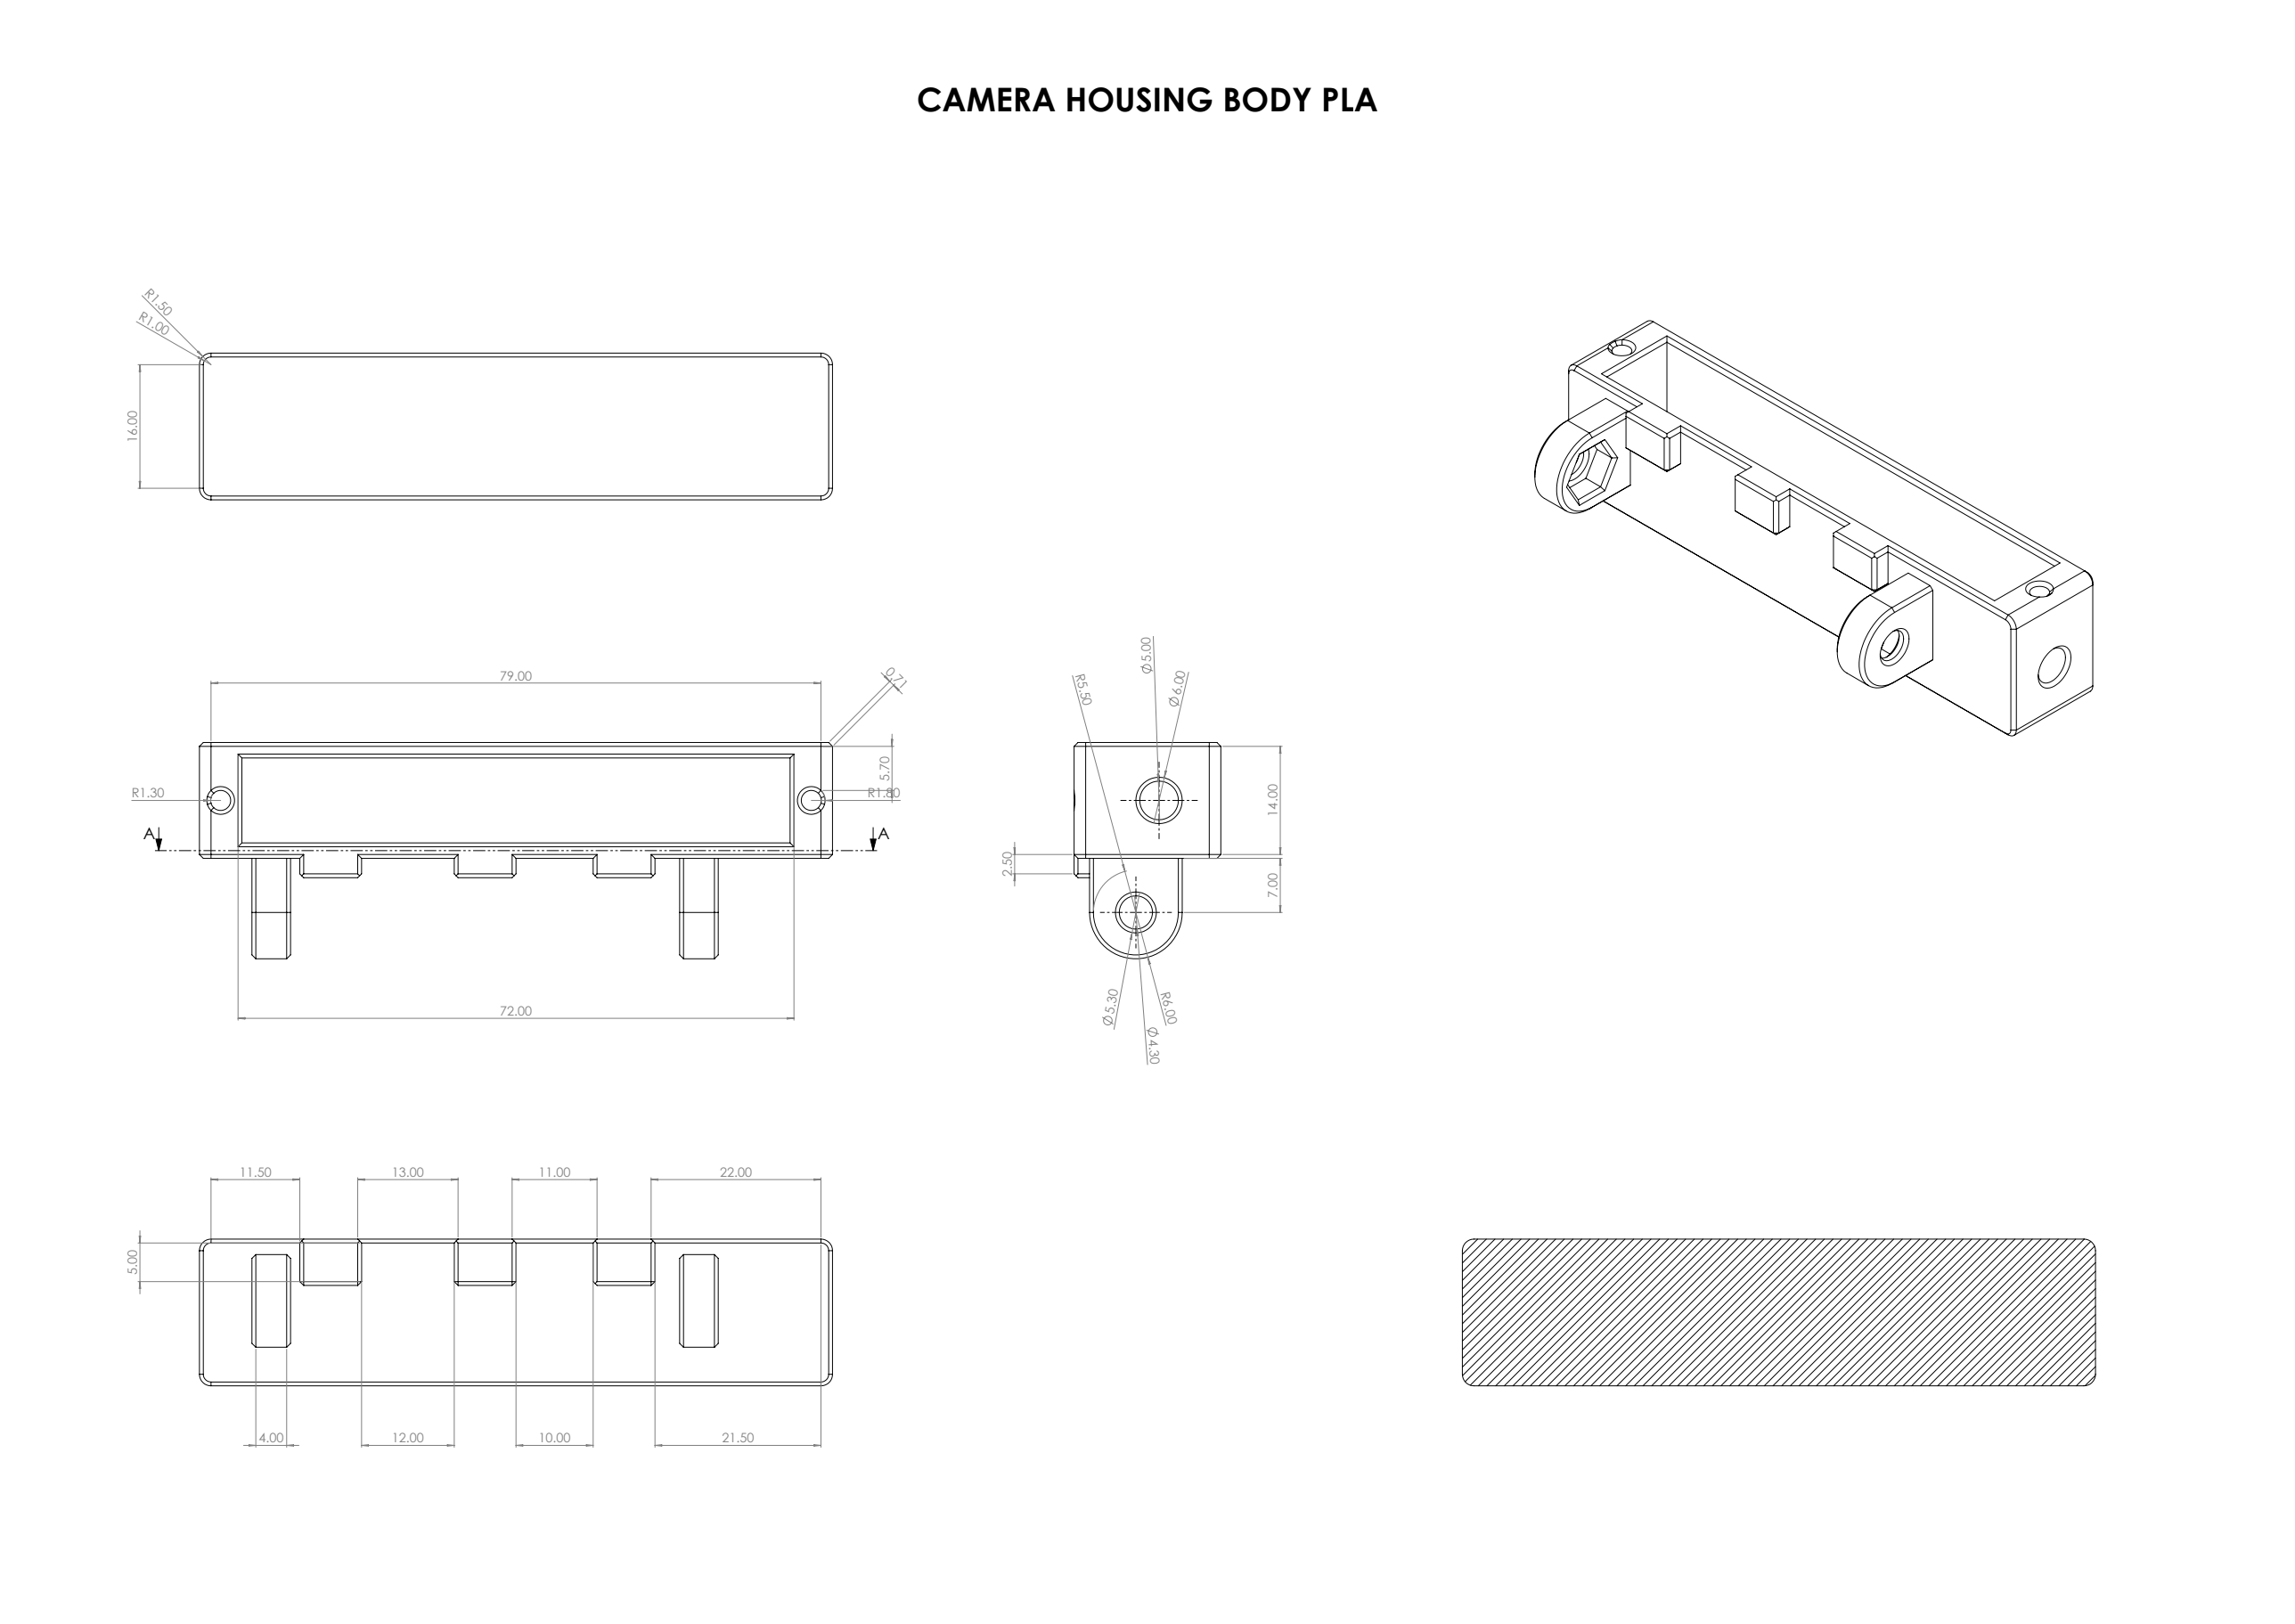
ISO-10303-21;
HEADER;
/* Generated by software containing ST-Developer
 * from STEP Tools, Inc. (www.steptools.com) 
 */

FILE_DESCRIPTION(
/* description */ (''),
/* implementation_level */ '2;1');

FILE_NAME(
/* name */ '03_Camera_Housing_Body_PLA.step',
/* time_stamp */ '2026-10-21T02:01:14-07:00',
/* author */ (''),
/* organization */ (''),
/* preprocessor_version */ 'ST-DEVELOPER v20.2',
/* originating_system */ 'Autodesk Translation Framework v15.15.0.0',
/* authorisation */ '');

FILE_SCHEMA (('AUTOMOTIVE_DESIGN { 1 0 10303 214 3 1 1 }'));
ENDSEC;

DATA;
#10=MECHANICAL_DESIGN_GEOMETRIC_PRESENTATION_REPRESENTATION('',(#616),#37181);
#105=B_SPLINE_SURFACE_WITH_KNOTS('',3,3,((#21181,#21182,#21183,#21184,#21185,
#21186),(#21187,#21188,#21189,#21190,#21191,#21192),(#21193,#21194,#21195,
#21196,#21197,#21198),(#21199,#21200,#21201,#21202,#21203,#21204)),
 .UNSPECIFIED.,.F.,.F.,.F.,(4,4),(4,2,4),(0.,1.),(0.268796457448958,0.30404357328347,
0.339290689117984),.UNSPECIFIED.);
#106=B_SPLINE_SURFACE_WITH_KNOTS('',3,3,((#21223,#21224,#21225,#21226),
(#21227,#21228,#21229,#21230),(#21231,#21232,#21233,#21234),(#21235,#21236,
#21237,#21238)),.UNSPECIFIED.,.F.,.F.,.F.,(4,4),(4,4),(0.,1.),(0.278246822734795,
0.803148805386868),.UNSPECIFIED.);
#107=B_SPLINE_SURFACE_WITH_KNOTS('',3,3,((#21243,#21244,#21245,#21246),
(#21247,#21248,#21249,#21250),(#21251,#21252,#21253,#21254),(#21255,#21256,
#21257,#21258)),.UNSPECIFIED.,.F.,.F.,.F.,(4,4),(4,4),(0.,1.),(-0.803148805386867,
-0.278246822734795),.UNSPECIFIED.);
#108=B_SPLINE_SURFACE_WITH_KNOTS('',3,3,((#21267,#21268,#21269,#21270,#21271,
#21272),(#21273,#21274,#21275,#21276,#21277,#21278),(#21279,#21280,#21281,
#21282,#21283,#21284),(#21285,#21286,#21287,#21288,#21289,#21290)),
 .UNSPECIFIED.,.F.,.F.,.F.,(4,4),(4,2,4),(0.,1.),(0.268796457448958,0.304043573283469,
0.33929068911798),.UNSPECIFIED.);
#109=B_SPLINE_SURFACE_WITH_KNOTS('',3,3,((#21310,#21311,#21312,#21313),
(#21314,#21315,#21316,#21317),(#21318,#21319,#21320,#21321),(#21322,#21323,
#21324,#21325)),.UNSPECIFIED.,.F.,.F.,.F.,(4,4),(4,4),(0.,1.),(-2.86334583085503,
-2.33844384820293),.UNSPECIFIED.);
#110=B_SPLINE_SURFACE_WITH_KNOTS('',3,3,((#21330,#21331,#21332,#21333),
(#21334,#21335,#21336,#21337),(#21338,#21339,#21340,#21341),(#21342,#21343,
#21344,#21345)),.UNSPECIFIED.,.F.,.F.,.F.,(4,4),(4,4),(0.,1.),(-3.94474145897665,
-3.41983947632457),.UNSPECIFIED.);
#128=B_SPLINE_CURVE_WITH_KNOTS('',3,(#21070,#21071,#21072,#21073),
 .UNSPECIFIED.,.F.,.F.,(4,4),(0.278246822734795,0.803148805386867),
 .UNSPECIFIED.);
#129=B_SPLINE_CURVE_WITH_KNOTS('',3,(#21075,#21076,#21077,#21078,#21079,
#21080),.UNSPECIFIED.,.F.,.F.,(4,2,4),(-0.339290689117984,-0.30404357328347,
-0.268796457448958),.UNSPECIFIED.);
#130=B_SPLINE_CURVE_WITH_KNOTS('',3,(#21081,#21082,#21083,#21084),
 .UNSPECIFIED.,.F.,.F.,(4,4),(-0.803148805386868,-0.278246822734795),
 .UNSPECIFIED.);
#131=B_SPLINE_CURVE_WITH_KNOTS('',3,(#21159,#21160,#21161,#21162),
 .UNSPECIFIED.,.F.,.F.,(4,4),(3.41983947632457,3.94474145897665),
 .UNSPECIFIED.);
#132=B_SPLINE_CURVE_WITH_KNOTS('',3,(#21164,#21165,#21166,#21167,#21168,
#21169),.UNSPECIFIED.,.F.,.F.,(4,2,4),(-0.33929068911798,-0.304043573283469,
-0.268796457448958),.UNSPECIFIED.);
#133=B_SPLINE_CURVE_WITH_KNOTS('',3,(#21170,#21171,#21172,#21173),
 .UNSPECIFIED.,.F.,.F.,(4,4),(2.33844384820293,2.86334583085503),
 .UNSPECIFIED.);
#134=B_SPLINE_CURVE_WITH_KNOTS('',3,(#21209,#21210,#21211,#21212,#21213,
#21214),.UNSPECIFIED.,.F.,.F.,(4,2,4),(0.268796457448958,0.30404357328347,
0.339290689117984),.UNSPECIFIED.);
#135=B_SPLINE_CURVE_WITH_KNOTS('',3,(#21239,#21240,#21241,#21242),
 .UNSPECIFIED.,.F.,.F.,(4,4),(0.278246822734795,0.803148805386868),
 .UNSPECIFIED.);
#136=B_SPLINE_CURVE_WITH_KNOTS('',3,(#21259,#21260,#21261,#21262),
 .UNSPECIFIED.,.F.,.F.,(4,4),(-0.803148805386867,-0.278246822734795),
 .UNSPECIFIED.);
#137=B_SPLINE_CURVE_WITH_KNOTS('',3,(#21296,#21297,#21298,#21299),
 .UNSPECIFIED.,.F.,.F.,(4,4),(0.268796457448958,0.304043573283469),
 .UNSPECIFIED.);
#138=B_SPLINE_CURVE_WITH_KNOTS('',3,(#21300,#21301,#21302,#21303),
 .UNSPECIFIED.,.F.,.F.,(4,4),(0.304043573283469,0.33929068911798),
 .UNSPECIFIED.);
#139=B_SPLINE_CURVE_WITH_KNOTS('',3,(#21326,#21327,#21328,#21329),
 .UNSPECIFIED.,.F.,.F.,(4,4),(-2.86334583085503,-2.33844384820293),
 .UNSPECIFIED.);
#140=B_SPLINE_CURVE_WITH_KNOTS('',3,(#21346,#21347,#21348,#21349),
 .UNSPECIFIED.,.F.,.F.,(4,4),(-3.94474145897665,-3.41983947632457),
 .UNSPECIFIED.);
#590=SHAPE_REPRESENTATION_RELATIONSHIP('SRR','None',#37240,#603);
#603=ADVANCED_BREP_SHAPE_REPRESENTATION('',(#629),#37170);
#616=STYLED_ITEM('',(#37352),#629);
#629=MANIFOLD_SOLID_BREP('Body1',#14778);
#654=FACE_BOUND('',#2365,.T.);
#655=FACE_BOUND('',#2382,.T.);
#656=FACE_BOUND('',#2386,.T.);
#657=FACE_BOUND('',#2389,.T.);
#658=FACE_BOUND('',#2401,.T.);
#659=FACE_BOUND('',#2415,.T.);
#660=FACE_BOUND('',#2446,.T.);
#661=FACE_BOUND('',#2457,.T.);
#662=FACE_BOUND('',#2484,.T.);
#663=FACE_BOUND('',#2485,.T.);
#664=FACE_BOUND('',#2502,.T.);
#708=CYLINDRICAL_SURFACE('',#15144,6.);
#709=CYLINDRICAL_SURFACE('',#15158,6.);
#710=CYLINDRICAL_SURFACE('',#15171,2.15);
#711=CYLINDRICAL_SURFACE('',#15177,2.15);
#712=CYLINDRICAL_SURFACE('',#15257,1.5);
#713=CYLINDRICAL_SURFACE('',#15261,1.5);
#714=CYLINDRICAL_SURFACE('',#15288,1.5);
#715=CYLINDRICAL_SURFACE('',#15290,1.5);
#716=CYLINDRICAL_SURFACE('',#15299,1.3);
#717=CYLINDRICAL_SURFACE('',#15303,1.3);
#718=CYLINDRICAL_SURFACE('',#15307,2.5);
#1019=CIRCLE('',#15140,5.5);
#1020=CIRCLE('',#15141,6.);
#1021=CIRCLE('',#15145,6.);
#1022=CIRCLE('',#15149,5.5);
#1023=CIRCLE('',#15154,5.5);
#1024=CIRCLE('',#15155,6.);
#1025=CIRCLE('',#15159,6.);
#1026=CIRCLE('',#15169,2.65);
#1027=CIRCLE('',#15170,2.15);
#1028=CIRCLE('',#15172,2.15);
#1029=CIRCLE('',#15175,2.65);
#1030=CIRCLE('',#15176,2.15);
#1031=CIRCLE('',#15178,2.15);
#1032=CIRCLE('',#15181,2.65);
#1033=CIRCLE('',#15193,2.65);
#1034=CIRCLE('',#15197,5.5);
#1035=CIRCLE('',#15239,1.8);
#1036=CIRCLE('',#15240,1.8);
#1037=CIRCLE('',#15243,1.5);
#1038=CIRCLE('',#15244,1.);
#1039=CIRCLE('',#15247,1.5);
#1040=CIRCLE('',#15248,1.);
#1041=CIRCLE('',#15251,1.5);
#1042=CIRCLE('',#15252,1.);
#1043=CIRCLE('',#15255,1.5);
#1044=CIRCLE('',#15256,1.);
#1045=CIRCLE('',#15258,1.5);
#1046=CIRCLE('',#15260,3.);
#1047=CIRCLE('',#15262,1.5);
#1048=CIRCLE('',#15269,1.5);
#1049=CIRCLE('',#15270,1.);
#1050=CIRCLE('',#15273,1.5);
#1051=CIRCLE('',#15274,1.);
#1052=CIRCLE('',#15277,1.);
#1053=CIRCLE('',#15280,1.);
#1054=CIRCLE('',#15297,1.3);
#1055=CIRCLE('',#15298,1.3);
#1056=CIRCLE('',#15300,1.3);
#1057=CIRCLE('',#15302,1.3);
#1058=CIRCLE('',#15304,1.3);
#1059=CIRCLE('',#15306,2.5);
#1060=CIRCLE('',#15308,2.5);
#1061=CIRCLE('',#15310,3.);
#1311=CONICAL_SURFACE('',#15139,5.75,0.785398163397448);
#1312=CONICAL_SURFACE('',#15148,5.75,0.785398163397448);
#1313=CONICAL_SURFACE('',#15153,5.75,0.785398163397448);
#1314=CONICAL_SURFACE('',#15168,2.4,0.785398163397448);
#1315=CONICAL_SURFACE('',#15174,2.4,0.785398163397448);
#1316=CONICAL_SURFACE('',#15180,2.4,0.785398163397448);
#1317=CONICAL_SURFACE('',#15192,2.4,0.785398163397448);
#1318=CONICAL_SURFACE('',#15196,5.75,0.785398163397448);
#1319=CONICAL_SURFACE('',#15242,1.25,0.785398163397451);
#1320=CONICAL_SURFACE('',#15246,1.25,0.785398163397449);
#1321=CONICAL_SURFACE('',#15250,1.25,0.785398163397449);
#1322=CONICAL_SURFACE('',#15254,1.25,0.785398163397451);
#1323=CONICAL_SURFACE('',#15268,1.25,0.785398163397451);
#1324=CONICAL_SURFACE('',#15272,1.25,0.785398163397449);
#1325=CONICAL_SURFACE('',#15276,1.25,0.785398163397449);
#1326=CONICAL_SURFACE('',#15279,1.25,0.785398163397451);
#1327=CONICAL_SURFACE('',#15296,1.55,0.785398163397446);
#1328=CONICAL_SURFACE('',#15301,1.55,0.785398163397446);
#1329=CONICAL_SURFACE('',#15305,2.75,0.785398163397448);
#1330=CONICAL_SURFACE('',#15309,2.75,0.785398163397448);
#1501=FACE_OUTER_BOUND('',#2355,.T.);
#1502=FACE_OUTER_BOUND('',#2356,.T.);
#1503=FACE_OUTER_BOUND('',#2357,.T.);
#1504=FACE_OUTER_BOUND('',#2358,.T.);
#1505=FACE_OUTER_BOUND('',#2359,.T.);
#1506=FACE_OUTER_BOUND('',#2360,.T.);
#1507=FACE_OUTER_BOUND('',#2361,.T.);
#1508=FACE_OUTER_BOUND('',#2362,.T.);
#1509=FACE_OUTER_BOUND('',#2363,.T.);
#1510=FACE_OUTER_BOUND('',#2364,.T.);
#1511=FACE_OUTER_BOUND('',#2366,.T.);
#1512=FACE_OUTER_BOUND('',#2367,.T.);
#1513=FACE_OUTER_BOUND('',#2368,.T.);
#1514=FACE_OUTER_BOUND('',#2369,.T.);
#1515=FACE_OUTER_BOUND('',#2370,.T.);
#1516=FACE_OUTER_BOUND('',#2371,.T.);
#1517=FACE_OUTER_BOUND('',#2372,.T.);
#1518=FACE_OUTER_BOUND('',#2373,.T.);
#1519=FACE_OUTER_BOUND('',#2374,.T.);
#1520=FACE_OUTER_BOUND('',#2375,.T.);
#1521=FACE_OUTER_BOUND('',#2376,.T.);
#1522=FACE_OUTER_BOUND('',#2377,.T.);
#1523=FACE_OUTER_BOUND('',#2378,.T.);
#1524=FACE_OUTER_BOUND('',#2379,.T.);
#1525=FACE_OUTER_BOUND('',#2380,.T.);
#1526=FACE_OUTER_BOUND('',#2381,.T.);
#1527=FACE_OUTER_BOUND('',#2383,.T.);
#1528=FACE_OUTER_BOUND('',#2384,.T.);
#1529=FACE_OUTER_BOUND('',#2385,.T.);
#1530=FACE_OUTER_BOUND('',#2387,.T.);
#1531=FACE_OUTER_BOUND('',#2388,.T.);
#1532=FACE_OUTER_BOUND('',#2390,.T.);
#1533=FACE_OUTER_BOUND('',#2391,.T.);
#1534=FACE_OUTER_BOUND('',#2392,.T.);
#1535=FACE_OUTER_BOUND('',#2393,.T.);
#1536=FACE_OUTER_BOUND('',#2394,.T.);
#1537=FACE_OUTER_BOUND('',#2395,.T.);
#1538=FACE_OUTER_BOUND('',#2396,.T.);
#1539=FACE_OUTER_BOUND('',#2397,.T.);
#1540=FACE_OUTER_BOUND('',#2398,.T.);
#1541=FACE_OUTER_BOUND('',#2399,.T.);
#1542=FACE_OUTER_BOUND('',#2400,.T.);
#1543=FACE_OUTER_BOUND('',#2402,.T.);
#1544=FACE_OUTER_BOUND('',#2403,.T.);
#1545=FACE_OUTER_BOUND('',#2404,.T.);
#1546=FACE_OUTER_BOUND('',#2405,.T.);
#1547=FACE_OUTER_BOUND('',#2406,.T.);
#1548=FACE_OUTER_BOUND('',#2407,.T.);
#1549=FACE_OUTER_BOUND('',#2408,.T.);
#1550=FACE_OUTER_BOUND('',#2409,.T.);
#1551=FACE_OUTER_BOUND('',#2410,.T.);
#1552=FACE_OUTER_BOUND('',#2411,.T.);
#1553=FACE_OUTER_BOUND('',#2412,.T.);
#1554=FACE_OUTER_BOUND('',#2413,.T.);
#1555=FACE_OUTER_BOUND('',#2414,.T.);
#1556=FACE_OUTER_BOUND('',#2416,.T.);
#1557=FACE_OUTER_BOUND('',#2417,.T.);
#1558=FACE_OUTER_BOUND('',#2418,.T.);
#1559=FACE_OUTER_BOUND('',#2419,.T.);
#1560=FACE_OUTER_BOUND('',#2420,.T.);
#1561=FACE_OUTER_BOUND('',#2421,.T.);
#1562=FACE_OUTER_BOUND('',#2422,.T.);
#1563=FACE_OUTER_BOUND('',#2423,.T.);
#1564=FACE_OUTER_BOUND('',#2424,.T.);
#1565=FACE_OUTER_BOUND('',#2425,.T.);
#1566=FACE_OUTER_BOUND('',#2426,.T.);
#1567=FACE_OUTER_BOUND('',#2427,.T.);
#1568=FACE_OUTER_BOUND('',#2428,.T.);
#1569=FACE_OUTER_BOUND('',#2429,.T.);
#1570=FACE_OUTER_BOUND('',#2430,.T.);
#1571=FACE_OUTER_BOUND('',#2431,.T.);
#1572=FACE_OUTER_BOUND('',#2432,.T.);
#1573=FACE_OUTER_BOUND('',#2433,.T.);
#1574=FACE_OUTER_BOUND('',#2434,.T.);
#1575=FACE_OUTER_BOUND('',#2435,.T.);
#1576=FACE_OUTER_BOUND('',#2436,.T.);
#1577=FACE_OUTER_BOUND('',#2437,.T.);
#1578=FACE_OUTER_BOUND('',#2438,.T.);
#1579=FACE_OUTER_BOUND('',#2439,.T.);
#1580=FACE_OUTER_BOUND('',#2440,.T.);
#1581=FACE_OUTER_BOUND('',#2441,.T.);
#1582=FACE_OUTER_BOUND('',#2442,.T.);
#1583=FACE_OUTER_BOUND('',#2443,.T.);
#1584=FACE_OUTER_BOUND('',#2444,.T.);
#1585=FACE_OUTER_BOUND('',#2445,.T.);
#1586=FACE_OUTER_BOUND('',#2447,.T.);
#1587=FACE_OUTER_BOUND('',#2448,.T.);
#1588=FACE_OUTER_BOUND('',#2449,.T.);
#1589=FACE_OUTER_BOUND('',#2450,.T.);
#1590=FACE_OUTER_BOUND('',#2451,.T.);
#1591=FACE_OUTER_BOUND('',#2452,.T.);
#1592=FACE_OUTER_BOUND('',#2453,.T.);
#1593=FACE_OUTER_BOUND('',#2454,.T.);
#1594=FACE_OUTER_BOUND('',#2455,.T.);
#1595=FACE_OUTER_BOUND('',#2456,.T.);
#1596=FACE_OUTER_BOUND('',#2458,.T.);
#1597=FACE_OUTER_BOUND('',#2459,.T.);
#1598=FACE_OUTER_BOUND('',#2460,.T.);
#1599=FACE_OUTER_BOUND('',#2461,.T.);
#1600=FACE_OUTER_BOUND('',#2462,.T.);
#1601=FACE_OUTER_BOUND('',#2463,.T.);
#1602=FACE_OUTER_BOUND('',#2464,.T.);
#1603=FACE_OUTER_BOUND('',#2465,.T.);
#1604=FACE_OUTER_BOUND('',#2466,.T.);
#1605=FACE_OUTER_BOUND('',#2467,.T.);
#1606=FACE_OUTER_BOUND('',#2468,.T.);
#1607=FACE_OUTER_BOUND('',#2469,.T.);
#1608=FACE_OUTER_BOUND('',#2470,.T.);
#1609=FACE_OUTER_BOUND('',#2471,.T.);
#1610=FACE_OUTER_BOUND('',#2472,.T.);
#1611=FACE_OUTER_BOUND('',#2473,.T.);
#1612=FACE_OUTER_BOUND('',#2474,.T.);
#1613=FACE_OUTER_BOUND('',#2475,.T.);
#1614=FACE_OUTER_BOUND('',#2476,.T.);
#1615=FACE_OUTER_BOUND('',#2477,.T.);
#1616=FACE_OUTER_BOUND('',#2478,.T.);
#1617=FACE_OUTER_BOUND('',#2479,.T.);
#1618=FACE_OUTER_BOUND('',#2480,.T.);
#1619=FACE_OUTER_BOUND('',#2481,.T.);
#1620=FACE_OUTER_BOUND('',#2482,.T.);
#1621=FACE_OUTER_BOUND('',#2483,.T.);
#1622=FACE_OUTER_BOUND('',#2486,.T.);
#1623=FACE_OUTER_BOUND('',#2487,.T.);
#1624=FACE_OUTER_BOUND('',#2488,.T.);
#1625=FACE_OUTER_BOUND('',#2489,.T.);
#1626=FACE_OUTER_BOUND('',#2490,.T.);
#1627=FACE_OUTER_BOUND('',#2491,.T.);
#1628=FACE_OUTER_BOUND('',#2492,.T.);
#1629=FACE_OUTER_BOUND('',#2493,.T.);
#1630=FACE_OUTER_BOUND('',#2494,.T.);
#1631=FACE_OUTER_BOUND('',#2495,.T.);
#1632=FACE_OUTER_BOUND('',#2496,.T.);
#1633=FACE_OUTER_BOUND('',#2497,.T.);
#1634=FACE_OUTER_BOUND('',#2498,.T.);
#1635=FACE_OUTER_BOUND('',#2499,.T.);
#1636=FACE_OUTER_BOUND('',#2500,.T.);
#1637=FACE_OUTER_BOUND('',#2501,.T.);
#1638=FACE_OUTER_BOUND('',#2503,.T.);
#1639=FACE_OUTER_BOUND('',#2504,.T.);
#1640=FACE_OUTER_BOUND('',#2505,.T.);
#1641=FACE_OUTER_BOUND('',#2506,.T.);
#1642=FACE_OUTER_BOUND('',#2507,.T.);
#1643=FACE_OUTER_BOUND('',#2508,.T.);
#1644=FACE_OUTER_BOUND('',#2509,.T.);
#1645=FACE_OUTER_BOUND('',#2510,.T.);
#1646=FACE_OUTER_BOUND('',#2511,.T.);
#1647=FACE_OUTER_BOUND('',#2512,.T.);
#1648=FACE_OUTER_BOUND('',#2513,.T.);
#2355=EDGE_LOOP('',(#9835,#9836,#9837,#9838));
#2356=EDGE_LOOP('',(#9839,#9840,#9841,#9842));
#2357=EDGE_LOOP('',(#9843,#9844,#9845,#9846));
#2358=EDGE_LOOP('',(#9847,#9848,#9849,#9850));
#2359=EDGE_LOOP('',(#9851,#9852,#9853,#9854));
#2360=EDGE_LOOP('',(#9855,#9856,#9857,#9858));
#2361=EDGE_LOOP('',(#9859,#9860,#9861,#9862));
#2362=EDGE_LOOP('',(#9863,#9864,#9865,#9866));
#2363=EDGE_LOOP('',(#9867,#9868,#9869,#9870));
#2364=EDGE_LOOP('',(#9871,#9872,#9873,#9874));
#2365=EDGE_LOOP('',(#9875,#9876,#9877,#9878,#9879,#9880));
#2366=EDGE_LOOP('',(#9881,#9882,#9883,#9884));
#2367=EDGE_LOOP('',(#9885,#9886,#9887,#9888));
#2368=EDGE_LOOP('',(#9889,#9890,#9891,#9892));
#2369=EDGE_LOOP('',(#9893,#9894,#9895,#9896));
#2370=EDGE_LOOP('',(#9897,#9898,#9899,#9900));
#2371=EDGE_LOOP('',(#9901,#9902,#9903,#9904));
#2372=EDGE_LOOP('',(#9905,#9906,#9907));
#2373=EDGE_LOOP('',(#9908,#9909,#9910,#9911));
#2374=EDGE_LOOP('',(#9912,#9913,#9914,#9915,#9916));
#2375=EDGE_LOOP('',(#9917,#9918,#9919,#9920,#9921));
#2376=EDGE_LOOP('',(#9922,#9923,#9924,#9925));
#2377=EDGE_LOOP('',(#9926,#9927,#9928,#9929));
#2378=EDGE_LOOP('',(#9930,#9931,#9932,#9933,#9934));
#2379=EDGE_LOOP('',(#9935,#9936,#9937,#9938));
#2380=EDGE_LOOP('',(#9939,#9940,#9941,#9942));
#2381=EDGE_LOOP('',(#9943,#9944,#9945,#9946));
#2382=EDGE_LOOP('',(#9947));
#2383=EDGE_LOOP('',(#9948,#9949,#9950,#9951));
#2384=EDGE_LOOP('',(#9952,#9953,#9954,#9955));
#2385=EDGE_LOOP('',(#9956,#9957,#9958,#9959));
#2386=EDGE_LOOP('',(#9960));
#2387=EDGE_LOOP('',(#9961,#9962,#9963,#9964));
#2388=EDGE_LOOP('',(#9965,#9966,#9967,#9968,#9969,#9970));
#2389=EDGE_LOOP('',(#9971));
#2390=EDGE_LOOP('',(#9972,#9973,#9974,#9975));
#2391=EDGE_LOOP('',(#9976,#9977,#9978,#9979));
#2392=EDGE_LOOP('',(#9980,#9981,#9982,#9983));
#2393=EDGE_LOOP('',(#9984,#9985,#9986,#9987));
#2394=EDGE_LOOP('',(#9988,#9989,#9990,#9991));
#2395=EDGE_LOOP('',(#9992,#9993,#9994,#9995));
#2396=EDGE_LOOP('',(#9996,#9997,#9998,#9999));
#2397=EDGE_LOOP('',(#10000,#10001,#10002,#10003));
#2398=EDGE_LOOP('',(#10004,#10005,#10006,#10007));
#2399=EDGE_LOOP('',(#10008,#10009,#10010,#10011));
#2400=EDGE_LOOP('',(#10012,#10013,#10014,#10015,#10016,#10017));
#2401=EDGE_LOOP('',(#10018));
#2402=EDGE_LOOP('',(#10019,#10020,#10021,#10022));
#2403=EDGE_LOOP('',(#10023,#10024,#10025,#10026));
#2404=EDGE_LOOP('',(#10027,#10028,#10029,#10030));
#2405=EDGE_LOOP('',(#10031,#10032,#10033,#10034));
#2406=EDGE_LOOP('',(#10035,#10036,#10037,#10038));
#2407=EDGE_LOOP('',(#10039,#10040,#10041,#10042));
#2408=EDGE_LOOP('',(#10043,#10044,#10045,#10046));
#2409=EDGE_LOOP('',(#10047,#10048,#10049,#10050));
#2410=EDGE_LOOP('',(#10051,#10052,#10053,#10054));
#2411=EDGE_LOOP('',(#10055,#10056,#10057,#10058));
#2412=EDGE_LOOP('',(#10059,#10060,#10061,#10062));
#2413=EDGE_LOOP('',(#10063,#10064,#10065,#10066));
#2414=EDGE_LOOP('',(#10067,#10068,#10069,#10070));
#2415=EDGE_LOOP('',(#10071,#10072,#10073,#10074,#10075,#10076));
#2416=EDGE_LOOP('',(#10077,#10078,#10079));
#2417=EDGE_LOOP('',(#10080,#10081,#10082,#10083));
#2418=EDGE_LOOP('',(#10084,#10085,#10086));
#2419=EDGE_LOOP('',(#10087,#10088,#10089,#10090));
#2420=EDGE_LOOP('',(#10091,#10092,#10093,#10094,#10095));
#2421=EDGE_LOOP('',(#10096,#10097,#10098,#10099));
#2422=EDGE_LOOP('',(#10100,#10101,#10102,#10103,#10104));
#2423=EDGE_LOOP('',(#10105,#10106,#10107,#10108));
#2424=EDGE_LOOP('',(#10109,#10110,#10111,#10112));
#2425=EDGE_LOOP('',(#10113,#10114,#10115,#10116,#10117));
#2426=EDGE_LOOP('',(#10118,#10119,#10120));
#2427=EDGE_LOOP('',(#10121,#10122,#10123,#10124));
#2428=EDGE_LOOP('',(#10125,#10126,#10127));
#2429=EDGE_LOOP('',(#10128,#10129,#10130,#10131));
#2430=EDGE_LOOP('',(#10132,#10133,#10134,#10135,#10136));
#2431=EDGE_LOOP('',(#10137,#10138,#10139,#10140));
#2432=EDGE_LOOP('',(#10141,#10142,#10143,#10144,#10145));
#2433=EDGE_LOOP('',(#10146,#10147,#10148,#10149));
#2434=EDGE_LOOP('',(#10150,#10151,#10152,#10153));
#2435=EDGE_LOOP('',(#10154,#10155,#10156,#10157,#10158));
#2436=EDGE_LOOP('',(#10159,#10160,#10161,#10162,#10163,#10164));
#2437=EDGE_LOOP('',(#10165,#10166,#10167,#10168));
#2438=EDGE_LOOP('',(#10169,#10170,#10171,#10172,#10173));
#2439=EDGE_LOOP('',(#10174,#10175,#10176,#10177));
#2440=EDGE_LOOP('',(#10178,#10179,#10180,#10181));
#2441=EDGE_LOOP('',(#10182,#10183,#10184,#10185));
#2442=EDGE_LOOP('',(#10186,#10187,#10188,#10189));
#2443=EDGE_LOOP('',(#10190,#10191,#10192,#10193));
#2444=EDGE_LOOP('',(#10194,#10195,#10196,#10197));
#2445=EDGE_LOOP('',(#10198,#10199,#10200,#10201,#10202,#10203,#10204,#10205,
#10206,#10207,#10208,#10209,#10210,#10211,#10212,#10213,#10214,#10215,#10216,
#10217));
#2446=EDGE_LOOP('',(#10218,#10219,#10220,#10221));
#2447=EDGE_LOOP('',(#10222,#10223,#10224,#10225));
#2448=EDGE_LOOP('',(#10226,#10227,#10228,#10229));
#2449=EDGE_LOOP('',(#10230,#10231,#10232,#10233));
#2450=EDGE_LOOP('',(#10234,#10235,#10236,#10237));
#2451=EDGE_LOOP('',(#10238,#10239,#10240,#10241));
#2452=EDGE_LOOP('',(#10242,#10243,#10244,#10245));
#2453=EDGE_LOOP('',(#10246,#10247,#10248,#10249));
#2454=EDGE_LOOP('',(#10250,#10251,#10252,#10253));
#2455=EDGE_LOOP('',(#10254,#10255,#10256,#10257));
#2456=EDGE_LOOP('',(#10258,#10259,#10260,#10261));
#2457=EDGE_LOOP('',(#10262));
#2458=EDGE_LOOP('',(#10263,#10264,#10265,#10266,#10267,#10268,#10269,#10270));
#2459=EDGE_LOOP('',(#10271,#10272,#10273,#10274,#10275,#10276,#10277,#10278));
#2460=EDGE_LOOP('',(#10279,#10280,#10281,#10282));
#2461=EDGE_LOOP('',(#10283,#10284,#10285,#10286));
#2462=EDGE_LOOP('',(#10287,#10288,#10289,#10290,#10291));
#2463=EDGE_LOOP('',(#10292,#10293,#10294,#10295));
#2464=EDGE_LOOP('',(#10296,#10297,#10298,#10299));
#2465=EDGE_LOOP('',(#10300,#10301,#10302,#10303));
#2466=EDGE_LOOP('',(#10304,#10305,#10306,#10307));
#2467=EDGE_LOOP('',(#10308,#10309,#10310,#10311));
#2468=EDGE_LOOP('',(#10312,#10313,#10314,#10315));
#2469=EDGE_LOOP('',(#10316,#10317,#10318,#10319));
#2470=EDGE_LOOP('',(#10320,#10321,#10322,#10323));
#2471=EDGE_LOOP('',(#10324,#10325,#10326,#10327));
#2472=EDGE_LOOP('',(#10328,#10329,#10330,#10331,#10332));
#2473=EDGE_LOOP('',(#10333,#10334,#10335,#10336,#10337,#10338));
#2474=EDGE_LOOP('',(#10339,#10340,#10341,#10342,#10343,#10344));
#2475=EDGE_LOOP('',(#10345,#10346,#10347,#10348,#10349));
#2476=EDGE_LOOP('',(#10350,#10351,#10352,#10353,#10354,#10355));
#2477=EDGE_LOOP('',(#10356,#10357,#10358,#10359));
#2478=EDGE_LOOP('',(#10360,#10361,#10362,#10363));
#2479=EDGE_LOOP('',(#10364,#10365,#10366,#10367));
#2480=EDGE_LOOP('',(#10368,#10369,#10370,#10371,#10372,#10373,#10374,#10375));
#2481=EDGE_LOOP('',(#10376,#10377,#10378,#10379));
#2482=EDGE_LOOP('',(#10380,#10381,#10382,#10383));
#2483=EDGE_LOOP('',(#10384,#10385,#10386,#10387,#10388,#10389,#10390,#10391,
#10392,#10393,#10394,#10395,#10396,#10397,#10398,#10399,#10400,#10401,#10402,
#10403,#10404,#10405,#10406,#10407,#10408,#10409));
#2484=EDGE_LOOP('',(#10410,#10411,#10412,#10413,#10414,#10415,#10416,#10417));
#2485=EDGE_LOOP('',(#10418,#10419,#10420,#10421,#10422,#10423,#10424,#10425));
#2486=EDGE_LOOP('',(#10426,#10427,#10428,#10429));
#2487=EDGE_LOOP('',(#10430,#10431,#10432,#10433));
#2488=EDGE_LOOP('',(#10434,#10435,#10436,#10437));
#2489=EDGE_LOOP('',(#10438,#10439,#10440,#10441,#10442));
#2490=EDGE_LOOP('',(#10443,#10444,#10445,#10446));
#2491=EDGE_LOOP('',(#10447,#10448,#10449,#10450));
#2492=EDGE_LOOP('',(#10451,#10452,#10453,#10454,#10455,#10456,#10457,#10458));
#2493=EDGE_LOOP('',(#10459,#10460,#10461,#10462,#10463));
#2494=EDGE_LOOP('',(#10464,#10465,#10466,#10467));
#2495=EDGE_LOOP('',(#10468,#10469,#10470,#10471));
#2496=EDGE_LOOP('',(#10472,#10473,#10474,#10475));
#2497=EDGE_LOOP('',(#10476,#10477,#10478,#10479,#10480,#10481,#10482,#10483));
#2498=EDGE_LOOP('',(#10484,#10485,#10486,#10487));
#2499=EDGE_LOOP('',(#10488,#10489,#10490,#10491));
#2500=EDGE_LOOP('',(#10492,#10493,#10494,#10495));
#2501=EDGE_LOOP('',(#10496,#10497,#10498,#10499));
#2502=EDGE_LOOP('',(#10500));
#2503=EDGE_LOOP('',(#10501));
#2504=EDGE_LOOP('',(#10502));
#2505=EDGE_LOOP('',(#10503,#10504,#10505,#10506));
#2506=EDGE_LOOP('',(#10507,#10508,#10509,#10510));
#2507=EDGE_LOOP('',(#10511,#10512,#10513,#10514));
#2508=EDGE_LOOP('',(#10515,#10516,#10517,#10518));
#2509=EDGE_LOOP('',(#10519,#10520,#10521,#10522));
#2510=EDGE_LOOP('',(#10523,#10524,#10525,#10526));
#2511=EDGE_LOOP('',(#10527,#10528,#10529,#10530));
#2512=EDGE_LOOP('',(#10531,#10532,#10533,#10534));
#2513=EDGE_LOOP('',(#10535,#10536,#10537,#10538));
#3419=LINE('',#20527,#4658);
#3420=LINE('',#20529,#4659);
#3421=LINE('',#20531,#4660);
#3422=LINE('',#20532,#4661);
#3423=LINE('',#20536,#4662);
#3424=LINE('',#20542,#4663);
#3425=LINE('',#20543,#4664);
#3426=LINE('',#20544,#4665);
#3427=LINE('',#20547,#4666);
#3428=LINE('',#20549,#4667);
#3429=LINE('',#20550,#4668);
#3430=LINE('',#20553,#4669);
#3431=LINE('',#20557,#4670);
#3432=LINE('',#20558,#4671);
#3433=LINE('',#20561,#4672);
#3434=LINE('',#20563,#4673);
#3435=LINE('',#20564,#4674);
#3436=LINE('',#20567,#4675);
#3437=LINE('',#20571,#4676);
#3438=LINE('',#20572,#4677);
#3439=LINE('',#20574,#4678);
#3440=LINE('',#20577,#4679);
#3441=LINE('',#20579,#4680);
#3442=LINE('',#20581,#4681);
#3443=LINE('',#20583,#4682);
#3444=LINE('',#20585,#4683);
#3445=LINE('',#20586,#4684);
#3446=LINE('',#20590,#4685);
#3447=LINE('',#20592,#4686);
#3448=LINE('',#20594,#4687);
#3449=LINE('',#20595,#4688);
#3450=LINE('',#20599,#4689);
#3451=LINE('',#20605,#4690);
#3452=LINE('',#20606,#4691);
#3453=LINE('',#20607,#4692);
#3454=LINE('',#20610,#4693);
#3455=LINE('',#20612,#4694);
#3456=LINE('',#20613,#4695);
#3457=LINE('',#20616,#4696);
#3458=LINE('',#20620,#4697);
#3459=LINE('',#20621,#4698);
#3460=LINE('',#20625,#4699);
#3461=LINE('',#20627,#4700);
#3462=LINE('',#20628,#4701);
#3463=LINE('',#20632,#4702);
#3464=LINE('',#20633,#4703);
#3465=LINE('',#20634,#4704);
#3466=LINE('',#20638,#4705);
#3467=LINE('',#20639,#4706);
#3468=LINE('',#20641,#4707);
#3469=LINE('',#20642,#4708);
#3470=LINE('',#20646,#4709);
#3471=LINE('',#20647,#4710);
#3472=LINE('',#20649,#4711);
#3473=LINE('',#20650,#4712);
#3474=LINE('',#20653,#4713);
#3475=LINE('',#20654,#4714);
#3476=LINE('',#20657,#4715);
#3477=LINE('',#20658,#4716);
#3478=LINE('',#20661,#4717);
#3479=LINE('',#20663,#4718);
#3480=LINE('',#20664,#4719);
#3481=LINE('',#20669,#4720);
#3482=LINE('',#20673,#4721);
#3483=LINE('',#20676,#4722);
#3484=LINE('',#20681,#4723);
#3485=LINE('',#20685,#4724);
#3486=LINE('',#20688,#4725);
#3487=LINE('',#20691,#4726);
#3488=LINE('',#20696,#4727);
#3489=LINE('',#20698,#4728);
#3490=LINE('',#20700,#4729);
#3491=LINE('',#20702,#4730);
#3492=LINE('',#20704,#4731);
#3493=LINE('',#20705,#4732);
#3494=LINE('',#20708,#4733);
#3495=LINE('',#20710,#4734);
#3496=LINE('',#20711,#4735);
#3497=LINE('',#20714,#4736);
#3498=LINE('',#20715,#4737);
#3499=LINE('',#20718,#4738);
#3500=LINE('',#20720,#4739);
#3501=LINE('',#20721,#4740);
#3502=LINE('',#20724,#4741);
#3503=LINE('',#20725,#4742);
#3504=LINE('',#20727,#4743);
#3505=LINE('',#20729,#4744);
#3506=LINE('',#20731,#4745);
#3507=LINE('',#20732,#4746);
#3508=LINE('',#20734,#4747);
#3509=LINE('',#20736,#4748);
#3510=LINE('',#20739,#4749);
#3511=LINE('',#20744,#4750);
#3512=LINE('',#20746,#4751);
#3513=LINE('',#20748,#4752);
#3514=LINE('',#20750,#4753);
#3515=LINE('',#20752,#4754);
#3516=LINE('',#20753,#4755);
#3517=LINE('',#20756,#4756);
#3518=LINE('',#20758,#4757);
#3519=LINE('',#20759,#4758);
#3520=LINE('',#20762,#4759);
#3521=LINE('',#20766,#4760);
#3522=LINE('',#20767,#4761);
#3523=LINE('',#20771,#4762);
#3524=LINE('',#20773,#4763);
#3525=LINE('',#20775,#4764);
#3526=LINE('',#20776,#4765);
#3527=LINE('',#20779,#4766);
#3528=LINE('',#20781,#4767);
#3529=LINE('',#20782,#4768);
#3530=LINE('',#20786,#4769);
#3531=LINE('',#20788,#4770);
#3532=LINE('',#20790,#4771);
#3533=LINE('',#20791,#4772);
#3534=LINE('',#20794,#4773);
#3535=LINE('',#20796,#4774);
#3536=LINE('',#20797,#4775);
#3537=LINE('',#20799,#4776);
#3538=LINE('',#20800,#4777);
#3539=LINE('',#20802,#4778);
#3540=LINE('',#20803,#4779);
#3541=LINE('',#20805,#4780);
#3542=LINE('',#20806,#4781);
#3543=LINE('',#20808,#4782);
#3544=LINE('',#20810,#4783);
#3545=LINE('',#20812,#4784);
#3546=LINE('',#20816,#4785);
#3547=LINE('',#20818,#4786);
#3548=LINE('',#20819,#4787);
#3549=LINE('',#20823,#4788);
#3550=LINE('',#20824,#4789);
#3551=LINE('',#20825,#4790);
#3552=LINE('',#20829,#4791);
#3553=LINE('',#20831,#4792);
#3554=LINE('',#20832,#4793);
#3555=LINE('',#20836,#4794);
#3556=LINE('',#20837,#4795);
#3557=LINE('',#20838,#4796);
#3558=LINE('',#20842,#4797);
#3559=LINE('',#20843,#4798);
#3560=LINE('',#20845,#4799);
#3561=LINE('',#20846,#4800);
#3562=LINE('',#20848,#4801);
#3563=LINE('',#20849,#4802);
#3564=LINE('',#20853,#4803);
#3565=LINE('',#20854,#4804);
#3566=LINE('',#20856,#4805);
#3567=LINE('',#20857,#4806);
#3568=LINE('',#20859,#4807);
#3569=LINE('',#20862,#4808);
#3570=LINE('',#20863,#4809);
#3571=LINE('',#20866,#4810);
#3572=LINE('',#20868,#4811);
#3573=LINE('',#20869,#4812);
#3574=LINE('',#20873,#4813);
#3575=LINE('',#20875,#4814);
#3576=LINE('',#20876,#4815);
#3577=LINE('',#20880,#4816);
#3578=LINE('',#20881,#4817);
#3579=LINE('',#20882,#4818);
#3580=LINE('',#20886,#4819);
#3581=LINE('',#20888,#4820);
#3582=LINE('',#20889,#4821);
#3583=LINE('',#20893,#4822);
#3584=LINE('',#20894,#4823);
#3585=LINE('',#20895,#4824);
#3586=LINE('',#20899,#4825);
#3587=LINE('',#20900,#4826);
#3588=LINE('',#20902,#4827);
#3589=LINE('',#20903,#4828);
#3590=LINE('',#20905,#4829);
#3591=LINE('',#20906,#4830);
#3592=LINE('',#20910,#4831);
#3593=LINE('',#20911,#4832);
#3594=LINE('',#20913,#4833);
#3595=LINE('',#20914,#4834);
#3596=LINE('',#20916,#4835);
#3597=LINE('',#20919,#4836);
#3598=LINE('',#20920,#4837);
#3599=LINE('',#20923,#4838);
#3600=LINE('',#20925,#4839);
#3601=LINE('',#20926,#4840);
#3602=LINE('',#20929,#4841);
#3603=LINE('',#20931,#4842);
#3604=LINE('',#20933,#4843);
#3605=LINE('',#20934,#4844);
#3606=LINE('',#20937,#4845);
#3607=LINE('',#20938,#4846);
#3608=LINE('',#20941,#4847);
#3609=LINE('',#20943,#4848);
#3610=LINE('',#20944,#4849);
#3611=LINE('',#20948,#4850);
#3612=LINE('',#20950,#4851);
#3613=LINE('',#20952,#4852);
#3614=LINE('',#20953,#4853);
#3615=LINE('',#20956,#4854);
#3616=LINE('',#20958,#4855);
#3617=LINE('',#20959,#4856);
#3618=LINE('',#20962,#4857);
#3619=LINE('',#20964,#4858);
#3620=LINE('',#20965,#4859);
#3621=LINE('',#20968,#4860);
#3622=LINE('',#20969,#4861);
#3623=LINE('',#20972,#4862);
#3624=LINE('',#20974,#4863);
#3625=LINE('',#20975,#4864);
#3626=LINE('',#20977,#4865);
#3627=LINE('',#20978,#4866);
#3628=LINE('',#20982,#4867);
#3629=LINE('',#20984,#4868);
#3630=LINE('',#20988,#4869);
#3631=LINE('',#20989,#4870);
#3632=LINE('',#20991,#4871);
#3633=LINE('',#20993,#4872);
#3634=LINE('',#20994,#4873);
#3635=LINE('',#20996,#4874);
#3636=LINE('',#20998,#4875);
#3637=LINE('',#20999,#4876);
#3638=LINE('',#21001,#4877);
#3639=LINE('',#21003,#4878);
#3640=LINE('',#21005,#4879);
#3641=LINE('',#21007,#4880);
#3642=LINE('',#21010,#4881);
#3643=LINE('',#21013,#4882);
#3644=LINE('',#21015,#4883);
#3645=LINE('',#21016,#4884);
#3646=LINE('',#21020,#4885);
#3647=LINE('',#21026,#4886);
#3648=LINE('',#21027,#4887);
#3649=LINE('',#21028,#4888);
#3650=LINE('',#21032,#4889);
#3651=LINE('',#21038,#4890);
#3652=LINE('',#21039,#4891);
#3653=LINE('',#21040,#4892);
#3654=LINE('',#21044,#4893);
#3655=LINE('',#21050,#4894);
#3656=LINE('',#21051,#4895);
#3657=LINE('',#21052,#4896);
#3658=LINE('',#21058,#4897);
#3659=LINE('',#21061,#4898);
#3660=LINE('',#21064,#4899);
#3661=LINE('',#21065,#4900);
#3662=LINE('',#21089,#4901);
#3663=LINE('',#21090,#4902);
#3664=LINE('',#21093,#4903);
#3665=LINE('',#21094,#4904);
#3666=LINE('',#21096,#4905);
#3667=LINE('',#21097,#4906);
#3668=LINE('',#21100,#4907);
#3669=LINE('',#21101,#4908);
#3670=LINE('',#21106,#4909);
#3671=LINE('',#21111,#4910);
#3672=LINE('',#21112,#4911);
#3673=LINE('',#21113,#4912);
#3674=LINE('',#21118,#4913);
#3675=LINE('',#21122,#4914);
#3676=LINE('',#21123,#4915);
#3677=LINE('',#21124,#4916);
#3678=LINE('',#21127,#4917);
#3679=LINE('',#21131,#4918);
#3680=LINE('',#21132,#4919);
#3681=LINE('',#21135,#4920);
#3682=LINE('',#21138,#4921);
#3683=LINE('',#21139,#4922);
#3684=LINE('',#21141,#4923);
#3685=LINE('',#21143,#4924);
#3686=LINE('',#21145,#4925);
#3687=LINE('',#21147,#4926);
#3688=LINE('',#21148,#4927);
#3689=LINE('',#21150,#4928);
#3690=LINE('',#21152,#4929);
#3691=LINE('',#21154,#4930);
#3692=LINE('',#21156,#4931);
#3693=LINE('',#21175,#4932);
#3694=LINE('',#21178,#4933);
#3695=LINE('',#21206,#4934);
#3696=LINE('',#21208,#4935);
#3697=LINE('',#21217,#4936);
#3698=LINE('',#21222,#4937);
#3699=LINE('',#21265,#4938);
#3700=LINE('',#21292,#4939);
#3701=LINE('',#21294,#4940);
#3702=LINE('',#21306,#4941);
#3703=LINE('',#21309,#4942);
#3704=LINE('',#21352,#4943);
#3705=LINE('',#21356,#4944);
#3706=LINE('',#21360,#4945);
#3707=LINE('',#21365,#4946);
#3708=LINE('',#21368,#4947);
#3709=LINE('',#21369,#4948);
#3710=LINE('',#21373,#4949);
#3711=LINE('',#21375,#4950);
#3712=LINE('',#21378,#4951);
#3713=LINE('',#21380,#4952);
#3714=LINE('',#21383,#4953);
#4658=VECTOR('',#16753,10.);
#4659=VECTOR('',#16754,10.);
#4660=VECTOR('',#16755,10.);
#4661=VECTOR('',#16756,10.);
#4662=VECTOR('',#16759,10.);
#4663=VECTOR('',#16766,10.);
#4664=VECTOR('',#16767,10.);
#4665=VECTOR('',#16768,10.);
#4666=VECTOR('',#16771,10.);
#4667=VECTOR('',#16772,10.);
#4668=VECTOR('',#16773,10.);
#4669=VECTOR('',#16776,10.);
#4670=VECTOR('',#16781,10.);
#4671=VECTOR('',#16782,10.);
#4672=VECTOR('',#16785,10.);
#4673=VECTOR('',#16786,10.);
#4674=VECTOR('',#16787,10.);
#4675=VECTOR('',#16790,10.);
#4676=VECTOR('',#16795,10.);
#4677=VECTOR('',#16796,10.);
#4678=VECTOR('',#16799,10.);
#4679=VECTOR('',#16800,10.);
#4680=VECTOR('',#16801,10.);
#4681=VECTOR('',#16802,10.);
#4682=VECTOR('',#16803,10.);
#4683=VECTOR('',#16804,10.);
#4684=VECTOR('',#16805,10.);
#4685=VECTOR('',#16808,10.);
#4686=VECTOR('',#16809,10.);
#4687=VECTOR('',#16810,10.);
#4688=VECTOR('',#16811,10.);
#4689=VECTOR('',#16814,10.);
#4690=VECTOR('',#16821,10.);
#4691=VECTOR('',#16822,10.);
#4692=VECTOR('',#16823,10.);
#4693=VECTOR('',#16826,10.);
#4694=VECTOR('',#16827,10.);
#4695=VECTOR('',#16828,10.);
#4696=VECTOR('',#16831,10.);
#4697=VECTOR('',#16836,10.);
#4698=VECTOR('',#16837,10.);
#4699=VECTOR('',#16840,10.);
#4700=VECTOR('',#16841,10.);
#4701=VECTOR('',#16842,10.);
#4702=VECTOR('',#16845,10.);
#4703=VECTOR('',#16846,10.);
#4704=VECTOR('',#16847,10.);
#4705=VECTOR('',#16850,10.);
#4706=VECTOR('',#16851,10.);
#4707=VECTOR('',#16852,10.);
#4708=VECTOR('',#16853,10.);
#4709=VECTOR('',#16856,10.);
#4710=VECTOR('',#16857,10.);
#4711=VECTOR('',#16858,10.);
#4712=VECTOR('',#16859,10.);
#4713=VECTOR('',#16862,10.);
#4714=VECTOR('',#16863,10.);
#4715=VECTOR('',#16866,10.);
#4716=VECTOR('',#16867,10.);
#4717=VECTOR('',#16870,10.);
#4718=VECTOR('',#16871,10.);
#4719=VECTOR('',#16872,10.);
#4720=VECTOR('',#16877,2.4);
#4721=VECTOR('',#16882,2.15);
#4722=VECTOR('',#16887,10.);
#4723=VECTOR('',#16892,2.4);
#4724=VECTOR('',#16897,2.15);
#4725=VECTOR('',#16902,10.);
#4726=VECTOR('',#16905,2.4);
#4727=VECTOR('',#16910,10.);
#4728=VECTOR('',#16911,10.);
#4729=VECTOR('',#16912,10.);
#4730=VECTOR('',#16913,10.);
#4731=VECTOR('',#16914,10.);
#4732=VECTOR('',#16915,10.);
#4733=VECTOR('',#16918,10.);
#4734=VECTOR('',#16919,10.);
#4735=VECTOR('',#16920,10.);
#4736=VECTOR('',#16923,10.);
#4737=VECTOR('',#16924,10.);
#4738=VECTOR('',#16927,10.);
#4739=VECTOR('',#16928,10.);
#4740=VECTOR('',#16929,10.);
#4741=VECTOR('',#16932,10.);
#4742=VECTOR('',#16933,10.);
#4743=VECTOR('',#16936,10.);
#4744=VECTOR('',#16939,10.);
#4745=VECTOR('',#16942,10.);
#4746=VECTOR('',#16943,10.);
#4747=VECTOR('',#16946,10.);
#4748=VECTOR('',#16949,10.);
#4749=VECTOR('',#16952,2.4);
#4750=VECTOR('',#16957,10.);
#4751=VECTOR('',#16958,10.);
#4752=VECTOR('',#16959,10.);
#4753=VECTOR('',#16960,10.);
#4754=VECTOR('',#16961,10.);
#4755=VECTOR('',#16962,10.);
#4756=VECTOR('',#16965,10.);
#4757=VECTOR('',#16966,10.);
#4758=VECTOR('',#16967,10.);
#4759=VECTOR('',#16970,10.);
#4760=VECTOR('',#16975,10.);
#4761=VECTOR('',#16976,10.);
#4762=VECTOR('',#16979,10.);
#4763=VECTOR('',#16980,10.);
#4764=VECTOR('',#16981,10.);
#4765=VECTOR('',#16982,10.);
#4766=VECTOR('',#16985,10.);
#4767=VECTOR('',#16986,10.);
#4768=VECTOR('',#16987,10.);
#4769=VECTOR('',#16990,10.);
#4770=VECTOR('',#16991,10.);
#4771=VECTOR('',#16992,10.);
#4772=VECTOR('',#16993,10.);
#4773=VECTOR('',#16996,10.);
#4774=VECTOR('',#16997,10.);
#4775=VECTOR('',#16998,10.);
#4776=VECTOR('',#17001,10.);
#4777=VECTOR('',#17002,10.);
#4778=VECTOR('',#17005,10.);
#4779=VECTOR('',#17006,10.);
#4780=VECTOR('',#17009,10.);
#4781=VECTOR('',#17010,10.);
#4782=VECTOR('',#17013,10.);
#4783=VECTOR('',#17016,10.);
#4784=VECTOR('',#17019,10.);
#4785=VECTOR('',#17022,10.);
#4786=VECTOR('',#17023,10.);
#4787=VECTOR('',#17024,10.);
#4788=VECTOR('',#17027,10.);
#4789=VECTOR('',#17028,10.);
#4790=VECTOR('',#17029,10.);
#4791=VECTOR('',#17032,10.);
#4792=VECTOR('',#17033,10.);
#4793=VECTOR('',#17034,10.);
#4794=VECTOR('',#17037,10.);
#4795=VECTOR('',#17038,10.);
#4796=VECTOR('',#17039,10.);
#4797=VECTOR('',#17042,10.);
#4798=VECTOR('',#17043,10.);
#4799=VECTOR('',#17044,10.);
#4800=VECTOR('',#17045,10.);
#4801=VECTOR('',#17048,10.);
#4802=VECTOR('',#17049,10.);
#4803=VECTOR('',#17052,10.);
#4804=VECTOR('',#17053,10.);
#4805=VECTOR('',#17054,10.);
#4806=VECTOR('',#17055,10.);
#4807=VECTOR('',#17058,10.);
#4808=VECTOR('',#17061,10.);
#4809=VECTOR('',#17062,10.);
#4810=VECTOR('',#17065,10.);
#4811=VECTOR('',#17066,10.);
#4812=VECTOR('',#17067,10.);
#4813=VECTOR('',#17070,10.);
#4814=VECTOR('',#17071,10.);
#4815=VECTOR('',#17072,10.);
#4816=VECTOR('',#17075,10.);
#4817=VECTOR('',#17076,10.);
#4818=VECTOR('',#17077,10.);
#4819=VECTOR('',#17080,10.);
#4820=VECTOR('',#17081,10.);
#4821=VECTOR('',#17082,10.);
#4822=VECTOR('',#17085,10.);
#4823=VECTOR('',#17086,10.);
#4824=VECTOR('',#17087,10.);
#4825=VECTOR('',#17090,10.);
#4826=VECTOR('',#17091,10.);
#4827=VECTOR('',#17092,10.);
#4828=VECTOR('',#17093,10.);
#4829=VECTOR('',#17096,10.);
#4830=VECTOR('',#17097,10.);
#4831=VECTOR('',#17100,10.);
#4832=VECTOR('',#17101,10.);
#4833=VECTOR('',#17102,10.);
#4834=VECTOR('',#17103,10.);
#4835=VECTOR('',#17106,10.);
#4836=VECTOR('',#17109,10.);
#4837=VECTOR('',#17110,10.);
#4838=VECTOR('',#17113,10.);
#4839=VECTOR('',#17114,10.);
#4840=VECTOR('',#17115,10.);
#4841=VECTOR('',#17118,10.);
#4842=VECTOR('',#17119,10.);
#4843=VECTOR('',#17120,10.);
#4844=VECTOR('',#17121,10.);
#4845=VECTOR('',#17124,10.);
#4846=VECTOR('',#17125,10.);
#4847=VECTOR('',#17128,10.);
#4848=VECTOR('',#17129,10.);
#4849=VECTOR('',#17130,10.);
#4850=VECTOR('',#17133,10.);
#4851=VECTOR('',#17134,10.);
#4852=VECTOR('',#17135,10.);
#4853=VECTOR('',#17136,10.);
#4854=VECTOR('',#17139,10.);
#4855=VECTOR('',#17140,10.);
#4856=VECTOR('',#17141,10.);
#4857=VECTOR('',#17144,10.);
#4858=VECTOR('',#17145,10.);
#4859=VECTOR('',#17146,10.);
#4860=VECTOR('',#17149,10.);
#4861=VECTOR('',#17150,10.);
#4862=VECTOR('',#17153,10.);
#4863=VECTOR('',#17154,10.);
#4864=VECTOR('',#17155,10.);
#4865=VECTOR('',#17158,10.);
#4866=VECTOR('',#17159,10.);
#4867=VECTOR('',#17162,10.);
#4868=VECTOR('',#17163,10.);
#4869=VECTOR('',#17166,10.);
#4870=VECTOR('',#17167,10.);
#4871=VECTOR('',#17168,10.);
#4872=VECTOR('',#17169,10.);
#4873=VECTOR('',#17170,10.);
#4874=VECTOR('',#17171,10.);
#4875=VECTOR('',#17172,10.);
#4876=VECTOR('',#17173,10.);
#4877=VECTOR('',#17174,10.);
#4878=VECTOR('',#17175,10.);
#4879=VECTOR('',#17176,10.);
#4880=VECTOR('',#17177,10.);
#4881=VECTOR('',#17180,10.);
#4882=VECTOR('',#17183,10.);
#4883=VECTOR('',#17184,10.);
#4884=VECTOR('',#17185,10.);
#4885=VECTOR('',#17188,10.);
#4886=VECTOR('',#17195,10.);
#4887=VECTOR('',#17196,10.);
#4888=VECTOR('',#17197,10.);
#4889=VECTOR('',#17200,10.);
#4890=VECTOR('',#17207,10.);
#4891=VECTOR('',#17208,10.);
#4892=VECTOR('',#17209,10.);
#4893=VECTOR('',#17212,10.);
#4894=VECTOR('',#17219,10.);
#4895=VECTOR('',#17220,10.);
#4896=VECTOR('',#17221,10.);
#4897=VECTOR('',#17230,10.);
#4898=VECTOR('',#17233,10.);
#4899=VECTOR('',#17236,10.);
#4900=VECTOR('',#17237,10.);
#4901=VECTOR('',#17248,10.);
#4902=VECTOR('',#17249,10.);
#4903=VECTOR('',#17252,10.);
#4904=VECTOR('',#17253,10.);
#4905=VECTOR('',#17256,10.);
#4906=VECTOR('',#17257,10.);
#4907=VECTOR('',#17260,10.);
#4908=VECTOR('',#17261,10.);
#4909=VECTOR('',#17266,10.);
#4910=VECTOR('',#17271,10.);
#4911=VECTOR('',#17272,10.);
#4912=VECTOR('',#17273,10.);
#4913=VECTOR('',#17278,10.);
#4914=VECTOR('',#17283,10.);
#4915=VECTOR('',#17284,10.);
#4916=VECTOR('',#17285,10.);
#4917=VECTOR('',#17288,10.);
#4918=VECTOR('',#17293,10.);
#4919=VECTOR('',#17294,10.);
#4920=VECTOR('',#17297,10.);
#4921=VECTOR('',#17302,10.);
#4922=VECTOR('',#17303,10.);
#4923=VECTOR('',#17306,10.);
#4924=VECTOR('',#17309,10.);
#4925=VECTOR('',#17312,10.);
#4926=VECTOR('',#17315,10.);
#4927=VECTOR('',#17316,10.);
#4928=VECTOR('',#17319,10.);
#4929=VECTOR('',#17322,10.);
#4930=VECTOR('',#17325,10.);
#4931=VECTOR('',#17328,10.);
#4932=VECTOR('',#17333,10.);
#4933=VECTOR('',#17338,10.);
#4934=VECTOR('',#17343,10.);
#4935=VECTOR('',#17344,10.);
#4936=VECTOR('',#17347,10.);
#4937=VECTOR('',#17352,10.);
#4938=VECTOR('',#17355,1.3);
#4939=VECTOR('',#17358,10.);
#4940=VECTOR('',#17359,10.);
#4941=VECTOR('',#17362,10.);
#4942=VECTOR('',#17365,10.);
#4943=VECTOR('',#17368,1.3);
#4944=VECTOR('',#17373,2.75);
#4945=VECTOR('',#17378,2.5);
#4946=VECTOR('',#17385,2.75);
#4947=VECTOR('',#17388,10.);
#4948=VECTOR('',#17389,10.);
#4949=VECTOR('',#17396,10.);
#4950=VECTOR('',#17399,10.);
#4951=VECTOR('',#17404,10.);
#4952=VECTOR('',#17407,10.);
#4953=VECTOR('',#17412,10.);
#5884=VERTEX_POINT('',#20525);
#5885=VERTEX_POINT('',#20526);
#5886=VERTEX_POINT('',#20528);
#5887=VERTEX_POINT('',#20530);
#5888=VERTEX_POINT('',#20534);
#5889=VERTEX_POINT('',#20535);
#5890=VERTEX_POINT('',#20540);
#5891=VERTEX_POINT('',#20541);
#5892=VERTEX_POINT('',#20546);
#5893=VERTEX_POINT('',#20548);
#5894=VERTEX_POINT('',#20552);
#5895=VERTEX_POINT('',#20556);
#5896=VERTEX_POINT('',#20560);
#5897=VERTEX_POINT('',#20562);
#5898=VERTEX_POINT('',#20566);
#5899=VERTEX_POINT('',#20570);
#5900=VERTEX_POINT('',#20575);
#5901=VERTEX_POINT('',#20576);
#5902=VERTEX_POINT('',#20578);
#5903=VERTEX_POINT('',#20580);
#5904=VERTEX_POINT('',#20582);
#5905=VERTEX_POINT('',#20584);
#5906=VERTEX_POINT('',#20588);
#5907=VERTEX_POINT('',#20589);
#5908=VERTEX_POINT('',#20591);
#5909=VERTEX_POINT('',#20593);
#5910=VERTEX_POINT('',#20597);
#5911=VERTEX_POINT('',#20598);
#5912=VERTEX_POINT('',#20603);
#5913=VERTEX_POINT('',#20604);
#5914=VERTEX_POINT('',#20609);
#5915=VERTEX_POINT('',#20611);
#5916=VERTEX_POINT('',#20615);
#5917=VERTEX_POINT('',#20619);
#5918=VERTEX_POINT('',#20623);
#5919=VERTEX_POINT('',#20624);
#5920=VERTEX_POINT('',#20626);
#5921=VERTEX_POINT('',#20630);
#5922=VERTEX_POINT('',#20631);
#5923=VERTEX_POINT('',#20636);
#5924=VERTEX_POINT('',#20637);
#5925=VERTEX_POINT('',#20640);
#5926=VERTEX_POINT('',#20644);
#5927=VERTEX_POINT('',#20645);
#5928=VERTEX_POINT('',#20648);
#5929=VERTEX_POINT('',#20652);
#5930=VERTEX_POINT('',#20656);
#5931=VERTEX_POINT('',#20660);
#5932=VERTEX_POINT('',#20662);
#5933=VERTEX_POINT('',#20666);
#5934=VERTEX_POINT('',#20668);
#5935=VERTEX_POINT('',#20672);
#5936=VERTEX_POINT('',#20678);
#5937=VERTEX_POINT('',#20680);
#5938=VERTEX_POINT('',#20684);
#5939=VERTEX_POINT('',#20690);
#5940=VERTEX_POINT('',#20694);
#5941=VERTEX_POINT('',#20695);
#5942=VERTEX_POINT('',#20697);
#5943=VERTEX_POINT('',#20699);
#5944=VERTEX_POINT('',#20701);
#5945=VERTEX_POINT('',#20703);
#5946=VERTEX_POINT('',#20707);
#5947=VERTEX_POINT('',#20709);
#5948=VERTEX_POINT('',#20713);
#5949=VERTEX_POINT('',#20717);
#5950=VERTEX_POINT('',#20719);
#5951=VERTEX_POINT('',#20723);
#5952=VERTEX_POINT('',#20738);
#5953=VERTEX_POINT('',#20742);
#5954=VERTEX_POINT('',#20743);
#5955=VERTEX_POINT('',#20745);
#5956=VERTEX_POINT('',#20747);
#5957=VERTEX_POINT('',#20749);
#5958=VERTEX_POINT('',#20751);
#5959=VERTEX_POINT('',#20755);
#5960=VERTEX_POINT('',#20757);
#5961=VERTEX_POINT('',#20761);
#5962=VERTEX_POINT('',#20765);
#5963=VERTEX_POINT('',#20769);
#5964=VERTEX_POINT('',#20770);
#5965=VERTEX_POINT('',#20772);
#5966=VERTEX_POINT('',#20774);
#5967=VERTEX_POINT('',#20778);
#5968=VERTEX_POINT('',#20780);
#5969=VERTEX_POINT('',#20784);
#5970=VERTEX_POINT('',#20785);
#5971=VERTEX_POINT('',#20787);
#5972=VERTEX_POINT('',#20789);
#5973=VERTEX_POINT('',#20793);
#5974=VERTEX_POINT('',#20795);
#5975=VERTEX_POINT('',#20814);
#5976=VERTEX_POINT('',#20815);
#5977=VERTEX_POINT('',#20817);
#5978=VERTEX_POINT('',#20821);
#5979=VERTEX_POINT('',#20822);
#5980=VERTEX_POINT('',#20827);
#5981=VERTEX_POINT('',#20828);
#5982=VERTEX_POINT('',#20830);
#5983=VERTEX_POINT('',#20834);
#5984=VERTEX_POINT('',#20835);
#5985=VERTEX_POINT('',#20840);
#5986=VERTEX_POINT('',#20841);
#5987=VERTEX_POINT('',#20844);
#5988=VERTEX_POINT('',#20851);
#5989=VERTEX_POINT('',#20852);
#5990=VERTEX_POINT('',#20855);
#5991=VERTEX_POINT('',#20861);
#5992=VERTEX_POINT('',#20865);
#5993=VERTEX_POINT('',#20867);
#5994=VERTEX_POINT('',#20871);
#5995=VERTEX_POINT('',#20872);
#5996=VERTEX_POINT('',#20874);
#5997=VERTEX_POINT('',#20878);
#5998=VERTEX_POINT('',#20879);
#5999=VERTEX_POINT('',#20884);
#6000=VERTEX_POINT('',#20885);
#6001=VERTEX_POINT('',#20887);
#6002=VERTEX_POINT('',#20891);
#6003=VERTEX_POINT('',#20892);
#6004=VERTEX_POINT('',#20897);
#6005=VERTEX_POINT('',#20898);
#6006=VERTEX_POINT('',#20901);
#6007=VERTEX_POINT('',#20908);
#6008=VERTEX_POINT('',#20909);
#6009=VERTEX_POINT('',#20912);
#6010=VERTEX_POINT('',#20918);
#6011=VERTEX_POINT('',#20922);
#6012=VERTEX_POINT('',#20924);
#6013=VERTEX_POINT('',#20928);
#6014=VERTEX_POINT('',#20930);
#6015=VERTEX_POINT('',#20932);
#6016=VERTEX_POINT('',#20936);
#6017=VERTEX_POINT('',#20940);
#6018=VERTEX_POINT('',#20942);
#6019=VERTEX_POINT('',#20946);
#6020=VERTEX_POINT('',#20947);
#6021=VERTEX_POINT('',#20949);
#6022=VERTEX_POINT('',#20951);
#6023=VERTEX_POINT('',#20955);
#6024=VERTEX_POINT('',#20957);
#6025=VERTEX_POINT('',#20961);
#6026=VERTEX_POINT('',#20963);
#6027=VERTEX_POINT('',#20967);
#6028=VERTEX_POINT('',#20971);
#6029=VERTEX_POINT('',#20973);
#6030=VERTEX_POINT('',#20980);
#6031=VERTEX_POINT('',#20981);
#6032=VERTEX_POINT('',#20983);
#6033=VERTEX_POINT('',#20985);
#6034=VERTEX_POINT('',#20987);
#6035=VERTEX_POINT('',#20990);
#6036=VERTEX_POINT('',#20992);
#6037=VERTEX_POINT('',#20995);
#6038=VERTEX_POINT('',#20997);
#6039=VERTEX_POINT('',#21000);
#6040=VERTEX_POINT('',#21002);
#6041=VERTEX_POINT('',#21004);
#6042=VERTEX_POINT('',#21006);
#6043=VERTEX_POINT('',#21008);
#6044=VERTEX_POINT('',#21012);
#6045=VERTEX_POINT('',#21014);
#6046=VERTEX_POINT('',#21018);
#6047=VERTEX_POINT('',#21019);
#6048=VERTEX_POINT('',#21024);
#6049=VERTEX_POINT('',#21025);
#6050=VERTEX_POINT('',#21030);
#6051=VERTEX_POINT('',#21031);
#6052=VERTEX_POINT('',#21036);
#6053=VERTEX_POINT('',#21037);
#6054=VERTEX_POINT('',#21042);
#6055=VERTEX_POINT('',#21043);
#6056=VERTEX_POINT('',#21048);
#6057=VERTEX_POINT('',#21049);
#6058=VERTEX_POINT('',#21057);
#6059=VERTEX_POINT('',#21059);
#6060=VERTEX_POINT('',#21063);
#6061=VERTEX_POINT('',#21066);
#6062=VERTEX_POINT('',#21069);
#6063=VERTEX_POINT('',#21074);
#6064=VERTEX_POINT('',#21088);
#6065=VERTEX_POINT('',#21092);
#6066=VERTEX_POINT('',#21099);
#6067=VERTEX_POINT('',#21103);
#6068=VERTEX_POINT('',#21105);
#6069=VERTEX_POINT('',#21109);
#6070=VERTEX_POINT('',#21110);
#6071=VERTEX_POINT('',#21115);
#6072=VERTEX_POINT('',#21117);
#6073=VERTEX_POINT('',#21121);
#6074=VERTEX_POINT('',#21126);
#6075=VERTEX_POINT('',#21130);
#6076=VERTEX_POINT('',#21134);
#6077=VERTEX_POINT('',#21158);
#6078=VERTEX_POINT('',#21163);
#6079=VERTEX_POINT('',#21205);
#6080=VERTEX_POINT('',#21207);
#6081=VERTEX_POINT('',#21216);
#6082=VERTEX_POINT('',#21218);
#6083=VERTEX_POINT('',#21220);
#6084=VERTEX_POINT('',#21264);
#6085=VERTEX_POINT('',#21291);
#6086=VERTEX_POINT('',#21293);
#6087=VERTEX_POINT('',#21295);
#6088=VERTEX_POINT('',#21305);
#6089=VERTEX_POINT('',#21307);
#6090=VERTEX_POINT('',#21351);
#6091=VERTEX_POINT('',#21355);
#6092=VERTEX_POINT('',#21359);
#6093=VERTEX_POINT('',#21363);
#6094=VERTEX_POINT('',#21367);
#7359=EDGE_CURVE('',#5884,#5885,#3419,.F.);
#7360=EDGE_CURVE('',#5885,#5886,#3420,.T.);
#7361=EDGE_CURVE('',#5886,#5887,#3421,.T.);
#7362=EDGE_CURVE('',#5887,#5884,#3422,.T.);
#7363=EDGE_CURVE('',#5888,#5889,#3423,.T.);
#7364=EDGE_CURVE('',#5889,#5887,#1019,.T.);
#7365=EDGE_CURVE('',#5886,#5888,#1020,.T.);
#7366=EDGE_CURVE('',#5890,#5891,#3424,.F.);
#7367=EDGE_CURVE('',#5891,#5889,#3425,.T.);
#7368=EDGE_CURVE('',#5888,#5890,#3426,.T.);
#7369=EDGE_CURVE('',#5892,#5888,#3427,.T.);
#7370=EDGE_CURVE('',#5893,#5892,#3428,.T.);
#7371=EDGE_CURVE('',#5890,#5893,#3429,.T.);
#7372=EDGE_CURVE('',#5894,#5886,#3430,.T.);
#7373=EDGE_CURVE('',#5892,#5894,#1021,.T.);
#7374=EDGE_CURVE('',#5895,#5885,#3431,.T.);
#7375=EDGE_CURVE('',#5894,#5895,#3432,.T.);
#7376=EDGE_CURVE('',#5895,#5896,#3433,.F.);
#7377=EDGE_CURVE('',#5896,#5897,#3434,.T.);
#7378=EDGE_CURVE('',#5897,#5894,#3435,.T.);
#7379=EDGE_CURVE('',#5898,#5892,#3436,.T.);
#7380=EDGE_CURVE('',#5897,#5898,#1022,.T.);
#7381=EDGE_CURVE('',#5899,#5893,#3437,.F.);
#7382=EDGE_CURVE('',#5898,#5899,#3438,.T.);
#7383=EDGE_CURVE('',#5899,#5896,#3439,.T.);
#7384=EDGE_CURVE('',#5900,#5901,#3440,.T.);
#7385=EDGE_CURVE('',#5902,#5900,#3441,.T.);
#7386=EDGE_CURVE('',#5903,#5902,#3442,.T.);
#7387=EDGE_CURVE('',#5904,#5903,#3443,.T.);
#7388=EDGE_CURVE('',#5905,#5904,#3444,.T.);
#7389=EDGE_CURVE('',#5901,#5905,#3445,.T.);
#7390=EDGE_CURVE('',#5906,#5907,#3446,.F.);
#7391=EDGE_CURVE('',#5907,#5908,#3447,.T.);
#7392=EDGE_CURVE('',#5908,#5909,#3448,.T.);
#7393=EDGE_CURVE('',#5909,#5906,#3449,.T.);
#7394=EDGE_CURVE('',#5910,#5911,#3450,.T.);
#7395=EDGE_CURVE('',#5911,#5909,#1023,.T.);
#7396=EDGE_CURVE('',#5908,#5910,#1024,.T.);
#7397=EDGE_CURVE('',#5912,#5913,#3451,.F.);
#7398=EDGE_CURVE('',#5913,#5911,#3452,.T.);
#7399=EDGE_CURVE('',#5910,#5912,#3453,.T.);
#7400=EDGE_CURVE('',#5914,#5910,#3454,.T.);
#7401=EDGE_CURVE('',#5915,#5914,#3455,.T.);
#7402=EDGE_CURVE('',#5912,#5915,#3456,.T.);
#7403=EDGE_CURVE('',#5916,#5908,#3457,.T.);
#7404=EDGE_CURVE('',#5914,#5916,#1025,.T.);
#7405=EDGE_CURVE('',#5917,#5907,#3458,.T.);
#7406=EDGE_CURVE('',#5916,#5917,#3459,.T.);
#7407=EDGE_CURVE('',#5918,#5919,#3460,.T.);
#7408=EDGE_CURVE('',#5920,#5918,#3461,.T.);
#7409=EDGE_CURVE('',#5919,#5920,#3462,.T.);
#7410=EDGE_CURVE('',#5921,#5922,#3463,.F.);
#7411=EDGE_CURVE('',#5922,#5920,#3464,.T.);
#7412=EDGE_CURVE('',#5918,#5921,#3465,.T.);
#7413=EDGE_CURVE('',#5923,#5924,#3466,.T.);
#7414=EDGE_CURVE('',#5924,#5919,#3467,.T.);
#7415=EDGE_CURVE('',#5920,#5925,#3468,.T.);
#7416=EDGE_CURVE('',#5925,#5923,#3469,.T.);
#7417=EDGE_CURVE('',#5926,#5927,#3470,.T.);
#7418=EDGE_CURVE('',#5927,#5918,#3471,.T.);
#7419=EDGE_CURVE('',#5919,#5928,#3472,.T.);
#7420=EDGE_CURVE('',#5928,#5926,#3473,.T.);
#7421=EDGE_CURVE('',#5929,#5922,#3474,.T.);
#7422=EDGE_CURVE('',#5925,#5929,#3475,.T.);
#7423=EDGE_CURVE('',#5930,#5927,#3476,.T.);
#7424=EDGE_CURVE('',#5921,#5930,#3477,.T.);
#7425=EDGE_CURVE('',#5926,#5931,#3478,.T.);
#7426=EDGE_CURVE('',#5931,#5932,#3479,.T.);
#7427=EDGE_CURVE('',#5932,#5930,#3480,.F.);
#7428=EDGE_CURVE('',#5933,#5933,#1026,.T.);
#7429=EDGE_CURVE('',#5933,#5934,#3481,.T.);
#7430=EDGE_CURVE('',#5934,#5934,#1027,.T.);
#7431=EDGE_CURVE('',#5934,#5935,#3482,.T.);
#7432=EDGE_CURVE('',#5935,#5935,#1028,.T.);
#7433=EDGE_CURVE('',#5884,#5891,#3483,.T.);
#7434=EDGE_CURVE('',#5936,#5936,#1029,.T.);
#7435=EDGE_CURVE('',#5936,#5937,#3484,.T.);
#7436=EDGE_CURVE('',#5937,#5937,#1030,.T.);
#7437=EDGE_CURVE('',#5937,#5938,#3485,.T.);
#7438=EDGE_CURVE('',#5938,#5938,#1031,.T.);
#7439=EDGE_CURVE('',#5906,#5913,#3486,.T.);
#7440=EDGE_CURVE('',#5935,#5939,#3487,.T.);
#7441=EDGE_CURVE('',#5939,#5939,#1032,.T.);
#7442=EDGE_CURVE('',#5940,#5941,#3488,.T.);
#7443=EDGE_CURVE('',#5942,#5940,#3489,.T.);
#7444=EDGE_CURVE('',#5943,#5942,#3490,.T.);
#7445=EDGE_CURVE('',#5944,#5943,#3491,.T.);
#7446=EDGE_CURVE('',#5945,#5944,#3492,.T.);
#7447=EDGE_CURVE('',#5941,#5945,#3493,.T.);
#7448=EDGE_CURVE('',#5903,#5946,#3494,.T.);
#7449=EDGE_CURVE('',#5946,#5947,#3495,.T.);
#7450=EDGE_CURVE('',#5904,#5947,#3496,.T.);
#7451=EDGE_CURVE('',#5902,#5948,#3497,.T.);
#7452=EDGE_CURVE('',#5948,#5946,#3498,.T.);
#7453=EDGE_CURVE('',#5901,#5949,#3499,.T.);
#7454=EDGE_CURVE('',#5949,#5950,#3500,.T.);
#7455=EDGE_CURVE('',#5950,#5900,#3501,.T.);
#7456=EDGE_CURVE('',#5951,#5949,#3502,.T.);
#7457=EDGE_CURVE('',#5905,#5951,#3503,.T.);
#7458=EDGE_CURVE('',#5950,#5948,#3504,.T.);
#7459=EDGE_CURVE('',#5947,#5951,#3505,.T.);
#7460=EDGE_CURVE('',#5948,#5941,#3506,.T.);
#7461=EDGE_CURVE('',#5946,#5945,#3507,.T.);
#7462=EDGE_CURVE('',#5950,#5940,#3508,.T.);
#7463=EDGE_CURVE('',#5949,#5942,#3509,.T.);
#7464=EDGE_CURVE('',#5938,#5952,#3510,.T.);
#7465=EDGE_CURVE('',#5952,#5952,#1033,.T.);
#7466=EDGE_CURVE('',#5953,#5954,#3511,.T.);
#7467=EDGE_CURVE('',#5955,#5953,#3512,.T.);
#7468=EDGE_CURVE('',#5956,#5955,#3513,.T.);
#7469=EDGE_CURVE('',#5957,#5956,#3514,.T.);
#7470=EDGE_CURVE('',#5958,#5957,#3515,.T.);
#7471=EDGE_CURVE('',#5954,#5958,#3516,.T.);
#7472=EDGE_CURVE('',#5959,#5915,#3517,.F.);
#7473=EDGE_CURVE('',#5914,#5960,#3518,.T.);
#7474=EDGE_CURVE('',#5960,#5959,#3519,.T.);
#7475=EDGE_CURVE('',#5916,#5961,#3520,.T.);
#7476=EDGE_CURVE('',#5961,#5960,#1034,.T.);
#7477=EDGE_CURVE('',#5917,#5962,#3521,.F.);
#7478=EDGE_CURVE('',#5962,#5961,#3522,.T.);
#7479=EDGE_CURVE('',#5963,#5964,#3523,.T.);
#7480=EDGE_CURVE('',#5964,#5965,#3524,.T.);
#7481=EDGE_CURVE('',#5965,#5966,#3525,.T.);
#7482=EDGE_CURVE('',#5963,#5966,#3526,.T.);
#7483=EDGE_CURVE('',#5964,#5967,#3527,.T.);
#7484=EDGE_CURVE('',#5967,#5968,#3528,.T.);
#7485=EDGE_CURVE('',#5968,#5965,#3529,.T.);
#7486=EDGE_CURVE('',#5969,#5970,#3530,.T.);
#7487=EDGE_CURVE('',#5970,#5971,#3531,.T.);
#7488=EDGE_CURVE('',#5971,#5972,#3532,.T.);
#7489=EDGE_CURVE('',#5972,#5969,#3533,.T.);
#7490=EDGE_CURVE('',#5973,#5971,#3534,.T.);
#7491=EDGE_CURVE('',#5970,#5974,#3535,.T.);
#7492=EDGE_CURVE('',#5974,#5973,#3536,.T.);
#7493=EDGE_CURVE('',#5967,#5969,#3537,.T.);
#7494=EDGE_CURVE('',#5972,#5968,#3538,.T.);
#7495=EDGE_CURVE('',#5966,#5973,#3539,.T.);
#7496=EDGE_CURVE('',#5974,#5963,#3540,.T.);
#7497=EDGE_CURVE('',#5968,#5954,#3541,.T.);
#7498=EDGE_CURVE('',#5965,#5958,#3542,.T.);
#7499=EDGE_CURVE('',#5972,#5953,#3543,.T.);
#7500=EDGE_CURVE('',#5971,#5955,#3544,.T.);
#7501=EDGE_CURVE('',#5959,#5962,#3545,.T.);
#7502=EDGE_CURVE('',#5975,#5976,#3546,.T.);
#7503=EDGE_CURVE('',#5977,#5975,#3547,.T.);
#7504=EDGE_CURVE('',#5976,#5977,#3548,.T.);
#7505=EDGE_CURVE('',#5978,#5979,#3549,.F.);
#7506=EDGE_CURVE('',#5979,#5977,#3550,.T.);
#7507=EDGE_CURVE('',#5975,#5978,#3551,.T.);
#7508=EDGE_CURVE('',#5980,#5981,#3552,.T.);
#7509=EDGE_CURVE('',#5982,#5980,#3553,.T.);
#7510=EDGE_CURVE('',#5981,#5982,#3554,.T.);
#7511=EDGE_CURVE('',#5983,#5984,#3555,.F.);
#7512=EDGE_CURVE('',#5984,#5982,#3556,.T.);
#7513=EDGE_CURVE('',#5980,#5983,#3557,.T.);
#7514=EDGE_CURVE('',#5985,#5986,#3558,.T.);
#7515=EDGE_CURVE('',#5986,#5981,#3559,.T.);
#7516=EDGE_CURVE('',#5982,#5987,#3560,.T.);
#7517=EDGE_CURVE('',#5987,#5985,#3561,.T.);
#7518=EDGE_CURVE('',#5981,#5976,#3562,.T.);
#7519=EDGE_CURVE('',#5977,#5980,#3563,.T.);
#7520=EDGE_CURVE('',#5988,#5989,#3564,.T.);
#7521=EDGE_CURVE('',#5989,#5975,#3565,.T.);
#7522=EDGE_CURVE('',#5976,#5990,#3566,.T.);
#7523=EDGE_CURVE('',#5990,#5988,#3567,.T.);
#7524=EDGE_CURVE('',#5983,#5979,#3568,.T.);
#7525=EDGE_CURVE('',#5991,#5989,#3569,.T.);
#7526=EDGE_CURVE('',#5978,#5991,#3570,.T.);
#7527=EDGE_CURVE('',#5988,#5992,#3571,.T.);
#7528=EDGE_CURVE('',#5992,#5993,#3572,.T.);
#7529=EDGE_CURVE('',#5991,#5993,#3573,.T.);
#7530=EDGE_CURVE('',#5994,#5995,#3574,.T.);
#7531=EDGE_CURVE('',#5996,#5994,#3575,.T.);
#7532=EDGE_CURVE('',#5995,#5996,#3576,.T.);
#7533=EDGE_CURVE('',#5997,#5998,#3577,.F.);
#7534=EDGE_CURVE('',#5998,#5996,#3578,.T.);
#7535=EDGE_CURVE('',#5994,#5997,#3579,.T.);
#7536=EDGE_CURVE('',#5999,#6000,#3580,.T.);
#7537=EDGE_CURVE('',#6001,#5999,#3581,.T.);
#7538=EDGE_CURVE('',#6000,#6001,#3582,.T.);
#7539=EDGE_CURVE('',#6002,#6003,#3583,.F.);
#7540=EDGE_CURVE('',#6003,#6001,#3584,.T.);
#7541=EDGE_CURVE('',#5999,#6002,#3585,.T.);
#7542=EDGE_CURVE('',#6004,#6005,#3586,.T.);
#7543=EDGE_CURVE('',#6005,#6000,#3587,.T.);
#7544=EDGE_CURVE('',#6001,#6006,#3588,.T.);
#7545=EDGE_CURVE('',#6006,#6004,#3589,.T.);
#7546=EDGE_CURVE('',#6000,#5995,#3590,.T.);
#7547=EDGE_CURVE('',#5996,#5999,#3591,.T.);
#7548=EDGE_CURVE('',#6007,#6008,#3592,.T.);
#7549=EDGE_CURVE('',#6008,#5994,#3593,.T.);
#7550=EDGE_CURVE('',#5995,#6009,#3594,.T.);
#7551=EDGE_CURVE('',#6009,#6007,#3595,.T.);
#7552=EDGE_CURVE('',#6002,#5998,#3596,.T.);
#7553=EDGE_CURVE('',#6010,#6008,#3597,.T.);
#7554=EDGE_CURVE('',#5997,#6010,#3598,.T.);
#7555=EDGE_CURVE('',#6007,#6011,#3599,.T.);
#7556=EDGE_CURVE('',#6011,#6012,#3600,.T.);
#7557=EDGE_CURVE('',#6010,#6012,#3601,.T.);
#7558=EDGE_CURVE('',#5928,#6013,#3602,.T.);
#7559=EDGE_CURVE('',#6013,#6014,#3603,.T.);
#7560=EDGE_CURVE('',#6014,#6015,#3604,.T.);
#7561=EDGE_CURVE('',#6015,#5931,#3605,.T.);
#7562=EDGE_CURVE('',#6016,#6015,#3606,.T.);
#7563=EDGE_CURVE('',#5932,#6016,#3607,.T.);
#7564=EDGE_CURVE('',#6014,#6017,#3608,.T.);
#7565=EDGE_CURVE('',#6017,#6018,#3609,.T.);
#7566=EDGE_CURVE('',#6016,#6018,#3610,.T.);
#7567=EDGE_CURVE('',#6019,#6020,#3611,.T.);
#7568=EDGE_CURVE('',#6020,#6021,#3612,.F.);
#7569=EDGE_CURVE('',#6021,#6022,#3613,.T.);
#7570=EDGE_CURVE('',#6022,#6019,#3614,.T.);
#7571=EDGE_CURVE('',#6022,#6023,#3615,.T.);
#7572=EDGE_CURVE('',#6023,#6024,#3616,.F.);
#7573=EDGE_CURVE('',#6024,#6019,#3617,.T.);
#7574=EDGE_CURVE('',#6019,#6025,#3618,.T.);
#7575=EDGE_CURVE('',#6025,#6026,#3619,.T.);
#7576=EDGE_CURVE('',#6020,#6026,#3620,.T.);
#7577=EDGE_CURVE('',#6024,#6027,#3621,.T.);
#7578=EDGE_CURVE('',#6027,#6025,#3622,.T.);
#7579=EDGE_CURVE('',#6028,#6021,#3623,.T.);
#7580=EDGE_CURVE('',#6020,#6029,#3624,.T.);
#7581=EDGE_CURVE('',#6029,#6028,#3625,.T.);
#7582=EDGE_CURVE('',#6029,#6024,#3626,.T.);
#7583=EDGE_CURVE('',#6023,#6028,#3627,.T.);
#7584=EDGE_CURVE('',#6030,#6031,#3628,.T.);
#7585=EDGE_CURVE('',#6032,#6030,#3629,.T.);
#7586=EDGE_CURVE('',#6033,#6032,#1035,.T.);
#7587=EDGE_CURVE('',#6034,#6033,#3630,.T.);
#7588=EDGE_CURVE('',#5993,#6034,#3631,.T.);
#7589=EDGE_CURVE('',#6035,#5992,#3632,.T.);
#7590=EDGE_CURVE('',#6036,#6035,#3633,.T.);
#7591=EDGE_CURVE('',#6012,#6036,#3634,.T.);
#7592=EDGE_CURVE('',#6037,#6011,#3635,.T.);
#7593=EDGE_CURVE('',#6038,#6037,#3636,.T.);
#7594=EDGE_CURVE('',#6018,#6038,#3637,.T.);
#7595=EDGE_CURVE('',#6039,#6017,#3638,.T.);
#7596=EDGE_CURVE('',#6040,#6039,#3639,.T.);
#7597=EDGE_CURVE('',#6041,#6040,#3640,.T.);
#7598=EDGE_CURVE('',#6042,#6041,#3641,.T.);
#7599=EDGE_CURVE('',#6043,#6042,#1036,.T.);
#7600=EDGE_CURVE('',#6031,#6043,#3642,.T.);
#7601=EDGE_CURVE('',#6044,#6030,#3643,.T.);
#7602=EDGE_CURVE('',#6031,#6045,#3644,.T.);
#7603=EDGE_CURVE('',#6045,#6044,#3645,.T.);
#7604=EDGE_CURVE('',#6046,#6047,#3646,.T.);
#7605=EDGE_CURVE('',#6047,#6030,#1037,.T.);
#7606=EDGE_CURVE('',#6044,#6046,#1038,.T.);
#7607=EDGE_CURVE('',#6048,#6049,#3647,.T.);
#7608=EDGE_CURVE('',#6049,#6047,#3648,.T.);
#7609=EDGE_CURVE('',#6046,#6048,#3649,.T.);
#7610=EDGE_CURVE('',#6050,#6051,#3650,.T.);
#7611=EDGE_CURVE('',#6051,#6049,#1039,.T.);
#7612=EDGE_CURVE('',#6048,#6050,#1040,.T.);
#7613=EDGE_CURVE('',#6052,#6053,#3651,.T.);
#7614=EDGE_CURVE('',#6053,#6051,#3652,.T.);
#7615=EDGE_CURVE('',#6050,#6052,#3653,.T.);
#7616=EDGE_CURVE('',#6054,#6055,#3654,.T.);
#7617=EDGE_CURVE('',#6055,#6053,#1041,.T.);
#7618=EDGE_CURVE('',#6052,#6054,#1042,.T.);
#7619=EDGE_CURVE('',#6056,#6057,#3655,.T.);
#7620=EDGE_CURVE('',#6057,#6055,#3656,.T.);
#7621=EDGE_CURVE('',#6054,#6056,#3657,.T.);
#7622=EDGE_CURVE('',#6031,#6057,#1043,.T.);
#7623=EDGE_CURVE('',#6056,#6045,#1044,.T.);
#7624=EDGE_CURVE('',#6055,#6058,#3658,.T.);
#7625=EDGE_CURVE('',#6059,#6058,#1045,.T.);
#7626=EDGE_CURVE('',#6059,#6053,#3659,.T.);
#7627=EDGE_CURVE('',#6060,#6057,#3660,.T.);
#7628=EDGE_CURVE('',#6058,#6060,#3661,.T.);
#7629=EDGE_CURVE('',#6061,#6061,#1046,.T.);
#7630=EDGE_CURVE('',#6062,#6043,#128,.T.);
#7631=EDGE_CURVE('',#6063,#6062,#129,.T.);
#7632=EDGE_CURVE('',#6042,#6063,#130,.T.);
#7633=EDGE_CURVE('',#6060,#6041,#1047,.T.);
#7634=EDGE_CURVE('',#6064,#6016,#3662,.T.);
#7635=EDGE_CURVE('',#6038,#6064,#3663,.T.);
#7636=EDGE_CURVE('',#6036,#6065,#3664,.T.);
#7637=EDGE_CURVE('',#6065,#6010,#3665,.T.);
#7638=EDGE_CURVE('',#5987,#6065,#3666,.T.);
#7639=EDGE_CURVE('',#6035,#5985,#3667,.T.);
#7640=EDGE_CURVE('',#6034,#6066,#3668,.T.);
#7641=EDGE_CURVE('',#6066,#5991,#3669,.T.);
#7642=EDGE_CURVE('',#6034,#6067,#1048,.T.);
#7643=EDGE_CURVE('',#6067,#6068,#3670,.T.);
#7644=EDGE_CURVE('',#6068,#6066,#1049,.T.);
#7645=EDGE_CURVE('',#6069,#6070,#3671,.T.);
#7646=EDGE_CURVE('',#6070,#6068,#3672,.T.);
#7647=EDGE_CURVE('',#6067,#6069,#3673,.T.);
#7648=EDGE_CURVE('',#6069,#6071,#1050,.T.);
#7649=EDGE_CURVE('',#6071,#6072,#3674,.T.);
#7650=EDGE_CURVE('',#6072,#6070,#1051,.T.);
#7651=EDGE_CURVE('',#6059,#6073,#3675,.T.);
#7652=EDGE_CURVE('',#6073,#6072,#3676,.T.);
#7653=EDGE_CURVE('',#6071,#6059,#3677,.T.);
#7654=EDGE_CURVE('',#6058,#6074,#3678,.T.);
#7655=EDGE_CURVE('',#6074,#6073,#1052,.T.);
#7656=EDGE_CURVE('',#6060,#6075,#3679,.T.);
#7657=EDGE_CURVE('',#6075,#6074,#3680,.T.);
#7658=EDGE_CURVE('',#6041,#6076,#3681,.T.);
#7659=EDGE_CURVE('',#6076,#6075,#1053,.T.);
#7660=EDGE_CURVE('',#5929,#6076,#3682,.T.);
#7661=EDGE_CURVE('',#6040,#5929,#3683,.T.);
#7662=EDGE_CURVE('',#6039,#5923,#3684,.T.);
#7663=EDGE_CURVE('',#5990,#5986,#3685,.T.);
#7664=EDGE_CURVE('',#6013,#5924,#3686,.T.);
#7665=EDGE_CURVE('',#6006,#6064,#3687,.T.);
#7666=EDGE_CURVE('',#6037,#6004,#3688,.T.);
#7667=EDGE_CURVE('',#6009,#6005,#3689,.T.);
#7668=EDGE_CURVE('',#6051,#6071,#3690,.T.);
#7669=EDGE_CURVE('',#6069,#6049,#3691,.T.);
#7670=EDGE_CURVE('',#6047,#6067,#3692,.T.);
#7671=EDGE_CURVE('',#6077,#6033,#131,.T.);
#7672=EDGE_CURVE('',#6078,#6077,#132,.T.);
#7673=EDGE_CURVE('',#6032,#6078,#133,.T.);
#7674=EDGE_CURVE('',#6064,#6003,#3693,.T.);
#7675=EDGE_CURVE('',#6065,#5984,#3694,.T.);
#7676=EDGE_CURVE('',#6079,#6063,#3695,.T.);
#7677=EDGE_CURVE('',#6062,#6080,#3696,.T.);
#7678=EDGE_CURVE('',#6080,#6079,#134,.T.);
#7679=EDGE_CURVE('',#6042,#6081,#3697,.T.);
#7680=EDGE_CURVE('',#6081,#6082,#1054,.T.);
#7681=EDGE_CURVE('',#6082,#6083,#1055,.T.);
#7682=EDGE_CURVE('',#6083,#6043,#3698,.T.);
#7683=EDGE_CURVE('',#6079,#6081,#135,.T.);
#7684=EDGE_CURVE('',#6083,#6080,#136,.T.);
#7685=EDGE_CURVE('',#6082,#6084,#3699,.T.);
#7686=EDGE_CURVE('',#6084,#6084,#1056,.T.);
#7687=EDGE_CURVE('',#6085,#6078,#3700,.T.);
#7688=EDGE_CURVE('',#6077,#6086,#3701,.T.);
#7689=EDGE_CURVE('',#6086,#6087,#137,.T.);
#7690=EDGE_CURVE('',#6087,#6085,#138,.T.);
#7691=EDGE_CURVE('',#6032,#6088,#3702,.T.);
#7692=EDGE_CURVE('',#6088,#6089,#1057,.T.);
#7693=EDGE_CURVE('',#6089,#6033,#3703,.T.);
#7694=EDGE_CURVE('',#6085,#6088,#139,.T.);
#7695=EDGE_CURVE('',#6089,#6086,#140,.T.);
#7696=EDGE_CURVE('',#6087,#6090,#3704,.T.);
#7697=EDGE_CURVE('',#6090,#6090,#1058,.T.);
#7698=EDGE_CURVE('',#6061,#6091,#3705,.T.);
#7699=EDGE_CURVE('',#6091,#6091,#1059,.T.);
#7700=EDGE_CURVE('',#6091,#6092,#3706,.T.);
#7701=EDGE_CURVE('',#6092,#6092,#1060,.T.);
#7702=EDGE_CURVE('',#6093,#6093,#1061,.T.);
#7703=EDGE_CURVE('',#6093,#6092,#3707,.T.);
#7704=EDGE_CURVE('',#6026,#6094,#3708,.T.);
#7705=EDGE_CURVE('',#6029,#6094,#3709,.T.);
#7706=EDGE_CURVE('',#5973,#5956,#3710,.T.);
#7707=EDGE_CURVE('',#5966,#5957,#3711,.T.);
#7708=EDGE_CURVE('',#5951,#5943,#3712,.T.);
#7709=EDGE_CURVE('',#5947,#5944,#3713,.T.);
#7710=EDGE_CURVE('',#6094,#6027,#3714,.T.);
#9835=ORIENTED_EDGE('',*,*,#7359,.T.);
#9836=ORIENTED_EDGE('',*,*,#7360,.T.);
#9837=ORIENTED_EDGE('',*,*,#7361,.T.);
#9838=ORIENTED_EDGE('',*,*,#7362,.T.);
#9839=ORIENTED_EDGE('',*,*,#7363,.T.);
#9840=ORIENTED_EDGE('',*,*,#7364,.T.);
#9841=ORIENTED_EDGE('',*,*,#7361,.F.);
#9842=ORIENTED_EDGE('',*,*,#7365,.T.);
#9843=ORIENTED_EDGE('',*,*,#7366,.T.);
#9844=ORIENTED_EDGE('',*,*,#7367,.T.);
#9845=ORIENTED_EDGE('',*,*,#7363,.F.);
#9846=ORIENTED_EDGE('',*,*,#7368,.T.);
#9847=ORIENTED_EDGE('',*,*,#7368,.F.);
#9848=ORIENTED_EDGE('',*,*,#7369,.F.);
#9849=ORIENTED_EDGE('',*,*,#7370,.F.);
#9850=ORIENTED_EDGE('',*,*,#7371,.F.);
#9851=ORIENTED_EDGE('',*,*,#7365,.F.);
#9852=ORIENTED_EDGE('',*,*,#7372,.F.);
#9853=ORIENTED_EDGE('',*,*,#7373,.F.);
#9854=ORIENTED_EDGE('',*,*,#7369,.T.);
#9855=ORIENTED_EDGE('',*,*,#7360,.F.);
#9856=ORIENTED_EDGE('',*,*,#7374,.F.);
#9857=ORIENTED_EDGE('',*,*,#7375,.F.);
#9858=ORIENTED_EDGE('',*,*,#7372,.T.);
#9859=ORIENTED_EDGE('',*,*,#7376,.T.);
#9860=ORIENTED_EDGE('',*,*,#7377,.T.);
#9861=ORIENTED_EDGE('',*,*,#7378,.T.);
#9862=ORIENTED_EDGE('',*,*,#7375,.T.);
#9863=ORIENTED_EDGE('',*,*,#7379,.T.);
#9864=ORIENTED_EDGE('',*,*,#7373,.T.);
#9865=ORIENTED_EDGE('',*,*,#7378,.F.);
#9866=ORIENTED_EDGE('',*,*,#7380,.T.);
#9867=ORIENTED_EDGE('',*,*,#7381,.T.);
#9868=ORIENTED_EDGE('',*,*,#7370,.T.);
#9869=ORIENTED_EDGE('',*,*,#7379,.F.);
#9870=ORIENTED_EDGE('',*,*,#7382,.T.);
#9871=ORIENTED_EDGE('',*,*,#7382,.F.);
#9872=ORIENTED_EDGE('',*,*,#7380,.F.);
#9873=ORIENTED_EDGE('',*,*,#7377,.F.);
#9874=ORIENTED_EDGE('',*,*,#7383,.F.);
#9875=ORIENTED_EDGE('',*,*,#7384,.F.);
#9876=ORIENTED_EDGE('',*,*,#7385,.F.);
#9877=ORIENTED_EDGE('',*,*,#7386,.F.);
#9878=ORIENTED_EDGE('',*,*,#7387,.F.);
#9879=ORIENTED_EDGE('',*,*,#7388,.F.);
#9880=ORIENTED_EDGE('',*,*,#7389,.F.);
#9881=ORIENTED_EDGE('',*,*,#7390,.T.);
#9882=ORIENTED_EDGE('',*,*,#7391,.T.);
#9883=ORIENTED_EDGE('',*,*,#7392,.T.);
#9884=ORIENTED_EDGE('',*,*,#7393,.T.);
#9885=ORIENTED_EDGE('',*,*,#7394,.T.);
#9886=ORIENTED_EDGE('',*,*,#7395,.T.);
#9887=ORIENTED_EDGE('',*,*,#7392,.F.);
#9888=ORIENTED_EDGE('',*,*,#7396,.T.);
#9889=ORIENTED_EDGE('',*,*,#7397,.T.);
#9890=ORIENTED_EDGE('',*,*,#7398,.T.);
#9891=ORIENTED_EDGE('',*,*,#7394,.F.);
#9892=ORIENTED_EDGE('',*,*,#7399,.T.);
#9893=ORIENTED_EDGE('',*,*,#7399,.F.);
#9894=ORIENTED_EDGE('',*,*,#7400,.F.);
#9895=ORIENTED_EDGE('',*,*,#7401,.F.);
#9896=ORIENTED_EDGE('',*,*,#7402,.F.);
#9897=ORIENTED_EDGE('',*,*,#7396,.F.);
#9898=ORIENTED_EDGE('',*,*,#7403,.F.);
#9899=ORIENTED_EDGE('',*,*,#7404,.F.);
#9900=ORIENTED_EDGE('',*,*,#7400,.T.);
#9901=ORIENTED_EDGE('',*,*,#7391,.F.);
#9902=ORIENTED_EDGE('',*,*,#7405,.F.);
#9903=ORIENTED_EDGE('',*,*,#7406,.F.);
#9904=ORIENTED_EDGE('',*,*,#7403,.T.);
#9905=ORIENTED_EDGE('',*,*,#7407,.F.);
#9906=ORIENTED_EDGE('',*,*,#7408,.F.);
#9907=ORIENTED_EDGE('',*,*,#7409,.F.);
#9908=ORIENTED_EDGE('',*,*,#7410,.T.);
#9909=ORIENTED_EDGE('',*,*,#7411,.T.);
#9910=ORIENTED_EDGE('',*,*,#7408,.T.);
#9911=ORIENTED_EDGE('',*,*,#7412,.T.);
#9912=ORIENTED_EDGE('',*,*,#7413,.T.);
#9913=ORIENTED_EDGE('',*,*,#7414,.T.);
#9914=ORIENTED_EDGE('',*,*,#7409,.T.);
#9915=ORIENTED_EDGE('',*,*,#7415,.T.);
#9916=ORIENTED_EDGE('',*,*,#7416,.T.);
#9917=ORIENTED_EDGE('',*,*,#7417,.T.);
#9918=ORIENTED_EDGE('',*,*,#7418,.T.);
#9919=ORIENTED_EDGE('',*,*,#7407,.T.);
#9920=ORIENTED_EDGE('',*,*,#7419,.T.);
#9921=ORIENTED_EDGE('',*,*,#7420,.T.);
#9922=ORIENTED_EDGE('',*,*,#7415,.F.);
#9923=ORIENTED_EDGE('',*,*,#7411,.F.);
#9924=ORIENTED_EDGE('',*,*,#7421,.F.);
#9925=ORIENTED_EDGE('',*,*,#7422,.F.);
#9926=ORIENTED_EDGE('',*,*,#7412,.F.);
#9927=ORIENTED_EDGE('',*,*,#7418,.F.);
#9928=ORIENTED_EDGE('',*,*,#7423,.F.);
#9929=ORIENTED_EDGE('',*,*,#7424,.F.);
#9930=ORIENTED_EDGE('',*,*,#7417,.F.);
#9931=ORIENTED_EDGE('',*,*,#7425,.T.);
#9932=ORIENTED_EDGE('',*,*,#7426,.T.);
#9933=ORIENTED_EDGE('',*,*,#7427,.T.);
#9934=ORIENTED_EDGE('',*,*,#7423,.T.);
#9935=ORIENTED_EDGE('',*,*,#7428,.T.);
#9936=ORIENTED_EDGE('',*,*,#7429,.T.);
#9937=ORIENTED_EDGE('',*,*,#7430,.T.);
#9938=ORIENTED_EDGE('',*,*,#7429,.F.);
#9939=ORIENTED_EDGE('',*,*,#7430,.F.);
#9940=ORIENTED_EDGE('',*,*,#7431,.T.);
#9941=ORIENTED_EDGE('',*,*,#7432,.F.);
#9942=ORIENTED_EDGE('',*,*,#7431,.F.);
#9943=ORIENTED_EDGE('',*,*,#7367,.F.);
#9944=ORIENTED_EDGE('',*,*,#7433,.F.);
#9945=ORIENTED_EDGE('',*,*,#7362,.F.);
#9946=ORIENTED_EDGE('',*,*,#7364,.F.);
#9947=ORIENTED_EDGE('',*,*,#7428,.F.);
#9948=ORIENTED_EDGE('',*,*,#7434,.T.);
#9949=ORIENTED_EDGE('',*,*,#7435,.T.);
#9950=ORIENTED_EDGE('',*,*,#7436,.T.);
#9951=ORIENTED_EDGE('',*,*,#7435,.F.);
#9952=ORIENTED_EDGE('',*,*,#7436,.F.);
#9953=ORIENTED_EDGE('',*,*,#7437,.T.);
#9954=ORIENTED_EDGE('',*,*,#7438,.F.);
#9955=ORIENTED_EDGE('',*,*,#7437,.F.);
#9956=ORIENTED_EDGE('',*,*,#7398,.F.);
#9957=ORIENTED_EDGE('',*,*,#7439,.F.);
#9958=ORIENTED_EDGE('',*,*,#7393,.F.);
#9959=ORIENTED_EDGE('',*,*,#7395,.F.);
#9960=ORIENTED_EDGE('',*,*,#7434,.F.);
#9961=ORIENTED_EDGE('',*,*,#7432,.T.);
#9962=ORIENTED_EDGE('',*,*,#7440,.T.);
#9963=ORIENTED_EDGE('',*,*,#7441,.T.);
#9964=ORIENTED_EDGE('',*,*,#7440,.F.);
#9965=ORIENTED_EDGE('',*,*,#7442,.F.);
#9966=ORIENTED_EDGE('',*,*,#7443,.F.);
#9967=ORIENTED_EDGE('',*,*,#7444,.F.);
#9968=ORIENTED_EDGE('',*,*,#7445,.F.);
#9969=ORIENTED_EDGE('',*,*,#7446,.F.);
#9970=ORIENTED_EDGE('',*,*,#7447,.F.);
#9971=ORIENTED_EDGE('',*,*,#7441,.F.);
#9972=ORIENTED_EDGE('',*,*,#7387,.T.);
#9973=ORIENTED_EDGE('',*,*,#7448,.T.);
#9974=ORIENTED_EDGE('',*,*,#7449,.T.);
#9975=ORIENTED_EDGE('',*,*,#7450,.F.);
#9976=ORIENTED_EDGE('',*,*,#7386,.T.);
#9977=ORIENTED_EDGE('',*,*,#7451,.T.);
#9978=ORIENTED_EDGE('',*,*,#7452,.T.);
#9979=ORIENTED_EDGE('',*,*,#7448,.F.);
#9980=ORIENTED_EDGE('',*,*,#7384,.T.);
#9981=ORIENTED_EDGE('',*,*,#7453,.T.);
#9982=ORIENTED_EDGE('',*,*,#7454,.T.);
#9983=ORIENTED_EDGE('',*,*,#7455,.T.);
#9984=ORIENTED_EDGE('',*,*,#7456,.T.);
#9985=ORIENTED_EDGE('',*,*,#7453,.F.);
#9986=ORIENTED_EDGE('',*,*,#7389,.T.);
#9987=ORIENTED_EDGE('',*,*,#7457,.T.);
#9988=ORIENTED_EDGE('',*,*,#7385,.T.);
#9989=ORIENTED_EDGE('',*,*,#7455,.F.);
#9990=ORIENTED_EDGE('',*,*,#7458,.T.);
#9991=ORIENTED_EDGE('',*,*,#7451,.F.);
#9992=ORIENTED_EDGE('',*,*,#7459,.T.);
#9993=ORIENTED_EDGE('',*,*,#7457,.F.);
#9994=ORIENTED_EDGE('',*,*,#7388,.T.);
#9995=ORIENTED_EDGE('',*,*,#7450,.T.);
#9996=ORIENTED_EDGE('',*,*,#7452,.F.);
#9997=ORIENTED_EDGE('',*,*,#7460,.T.);
#9998=ORIENTED_EDGE('',*,*,#7447,.T.);
#9999=ORIENTED_EDGE('',*,*,#7461,.F.);
#10000=ORIENTED_EDGE('',*,*,#7458,.F.);
#10001=ORIENTED_EDGE('',*,*,#7462,.T.);
#10002=ORIENTED_EDGE('',*,*,#7442,.T.);
#10003=ORIENTED_EDGE('',*,*,#7460,.F.);
#10004=ORIENTED_EDGE('',*,*,#7454,.F.);
#10005=ORIENTED_EDGE('',*,*,#7463,.T.);
#10006=ORIENTED_EDGE('',*,*,#7443,.T.);
#10007=ORIENTED_EDGE('',*,*,#7462,.F.);
#10008=ORIENTED_EDGE('',*,*,#7438,.T.);
#10009=ORIENTED_EDGE('',*,*,#7464,.T.);
#10010=ORIENTED_EDGE('',*,*,#7465,.T.);
#10011=ORIENTED_EDGE('',*,*,#7464,.F.);
#10012=ORIENTED_EDGE('',*,*,#7466,.F.);
#10013=ORIENTED_EDGE('',*,*,#7467,.F.);
#10014=ORIENTED_EDGE('',*,*,#7468,.F.);
#10015=ORIENTED_EDGE('',*,*,#7469,.F.);
#10016=ORIENTED_EDGE('',*,*,#7470,.F.);
#10017=ORIENTED_EDGE('',*,*,#7471,.F.);
#10018=ORIENTED_EDGE('',*,*,#7465,.F.);
#10019=ORIENTED_EDGE('',*,*,#7472,.T.);
#10020=ORIENTED_EDGE('',*,*,#7401,.T.);
#10021=ORIENTED_EDGE('',*,*,#7473,.T.);
#10022=ORIENTED_EDGE('',*,*,#7474,.T.);
#10023=ORIENTED_EDGE('',*,*,#7475,.T.);
#10024=ORIENTED_EDGE('',*,*,#7476,.T.);
#10025=ORIENTED_EDGE('',*,*,#7473,.F.);
#10026=ORIENTED_EDGE('',*,*,#7404,.T.);
#10027=ORIENTED_EDGE('',*,*,#7477,.T.);
#10028=ORIENTED_EDGE('',*,*,#7478,.T.);
#10029=ORIENTED_EDGE('',*,*,#7475,.F.);
#10030=ORIENTED_EDGE('',*,*,#7406,.T.);
#10031=ORIENTED_EDGE('',*,*,#7479,.T.);
#10032=ORIENTED_EDGE('',*,*,#7480,.T.);
#10033=ORIENTED_EDGE('',*,*,#7481,.T.);
#10034=ORIENTED_EDGE('',*,*,#7482,.F.);
#10035=ORIENTED_EDGE('',*,*,#7483,.T.);
#10036=ORIENTED_EDGE('',*,*,#7484,.T.);
#10037=ORIENTED_EDGE('',*,*,#7485,.T.);
#10038=ORIENTED_EDGE('',*,*,#7480,.F.);
#10039=ORIENTED_EDGE('',*,*,#7486,.T.);
#10040=ORIENTED_EDGE('',*,*,#7487,.T.);
#10041=ORIENTED_EDGE('',*,*,#7488,.T.);
#10042=ORIENTED_EDGE('',*,*,#7489,.T.);
#10043=ORIENTED_EDGE('',*,*,#7490,.T.);
#10044=ORIENTED_EDGE('',*,*,#7487,.F.);
#10045=ORIENTED_EDGE('',*,*,#7491,.T.);
#10046=ORIENTED_EDGE('',*,*,#7492,.T.);
#10047=ORIENTED_EDGE('',*,*,#7493,.T.);
#10048=ORIENTED_EDGE('',*,*,#7489,.F.);
#10049=ORIENTED_EDGE('',*,*,#7494,.T.);
#10050=ORIENTED_EDGE('',*,*,#7484,.F.);
#10051=ORIENTED_EDGE('',*,*,#7495,.T.);
#10052=ORIENTED_EDGE('',*,*,#7492,.F.);
#10053=ORIENTED_EDGE('',*,*,#7496,.T.);
#10054=ORIENTED_EDGE('',*,*,#7482,.T.);
#10055=ORIENTED_EDGE('',*,*,#7485,.F.);
#10056=ORIENTED_EDGE('',*,*,#7497,.T.);
#10057=ORIENTED_EDGE('',*,*,#7471,.T.);
#10058=ORIENTED_EDGE('',*,*,#7498,.F.);
#10059=ORIENTED_EDGE('',*,*,#7494,.F.);
#10060=ORIENTED_EDGE('',*,*,#7499,.T.);
#10061=ORIENTED_EDGE('',*,*,#7466,.T.);
#10062=ORIENTED_EDGE('',*,*,#7497,.F.);
#10063=ORIENTED_EDGE('',*,*,#7488,.F.);
#10064=ORIENTED_EDGE('',*,*,#7500,.T.);
#10065=ORIENTED_EDGE('',*,*,#7467,.T.);
#10066=ORIENTED_EDGE('',*,*,#7499,.F.);
#10067=ORIENTED_EDGE('',*,*,#7478,.F.);
#10068=ORIENTED_EDGE('',*,*,#7501,.F.);
#10069=ORIENTED_EDGE('',*,*,#7474,.F.);
#10070=ORIENTED_EDGE('',*,*,#7476,.F.);
#10071=ORIENTED_EDGE('',*,*,#7486,.F.);
#10072=ORIENTED_EDGE('',*,*,#7493,.F.);
#10073=ORIENTED_EDGE('',*,*,#7483,.F.);
#10074=ORIENTED_EDGE('',*,*,#7479,.F.);
#10075=ORIENTED_EDGE('',*,*,#7496,.F.);
#10076=ORIENTED_EDGE('',*,*,#7491,.F.);
#10077=ORIENTED_EDGE('',*,*,#7502,.F.);
#10078=ORIENTED_EDGE('',*,*,#7503,.F.);
#10079=ORIENTED_EDGE('',*,*,#7504,.F.);
#10080=ORIENTED_EDGE('',*,*,#7505,.T.);
#10081=ORIENTED_EDGE('',*,*,#7506,.T.);
#10082=ORIENTED_EDGE('',*,*,#7503,.T.);
#10083=ORIENTED_EDGE('',*,*,#7507,.T.);
#10084=ORIENTED_EDGE('',*,*,#7508,.F.);
#10085=ORIENTED_EDGE('',*,*,#7509,.F.);
#10086=ORIENTED_EDGE('',*,*,#7510,.F.);
#10087=ORIENTED_EDGE('',*,*,#7511,.T.);
#10088=ORIENTED_EDGE('',*,*,#7512,.T.);
#10089=ORIENTED_EDGE('',*,*,#7509,.T.);
#10090=ORIENTED_EDGE('',*,*,#7513,.T.);
#10091=ORIENTED_EDGE('',*,*,#7514,.T.);
#10092=ORIENTED_EDGE('',*,*,#7515,.T.);
#10093=ORIENTED_EDGE('',*,*,#7510,.T.);
#10094=ORIENTED_EDGE('',*,*,#7516,.T.);
#10095=ORIENTED_EDGE('',*,*,#7517,.T.);
#10096=ORIENTED_EDGE('',*,*,#7508,.T.);
#10097=ORIENTED_EDGE('',*,*,#7518,.T.);
#10098=ORIENTED_EDGE('',*,*,#7504,.T.);
#10099=ORIENTED_EDGE('',*,*,#7519,.T.);
#10100=ORIENTED_EDGE('',*,*,#7520,.T.);
#10101=ORIENTED_EDGE('',*,*,#7521,.T.);
#10102=ORIENTED_EDGE('',*,*,#7502,.T.);
#10103=ORIENTED_EDGE('',*,*,#7522,.T.);
#10104=ORIENTED_EDGE('',*,*,#7523,.T.);
#10105=ORIENTED_EDGE('',*,*,#7513,.F.);
#10106=ORIENTED_EDGE('',*,*,#7519,.F.);
#10107=ORIENTED_EDGE('',*,*,#7506,.F.);
#10108=ORIENTED_EDGE('',*,*,#7524,.F.);
#10109=ORIENTED_EDGE('',*,*,#7507,.F.);
#10110=ORIENTED_EDGE('',*,*,#7521,.F.);
#10111=ORIENTED_EDGE('',*,*,#7525,.F.);
#10112=ORIENTED_EDGE('',*,*,#7526,.F.);
#10113=ORIENTED_EDGE('',*,*,#7520,.F.);
#10114=ORIENTED_EDGE('',*,*,#7527,.T.);
#10115=ORIENTED_EDGE('',*,*,#7528,.T.);
#10116=ORIENTED_EDGE('',*,*,#7529,.F.);
#10117=ORIENTED_EDGE('',*,*,#7525,.T.);
#10118=ORIENTED_EDGE('',*,*,#7530,.F.);
#10119=ORIENTED_EDGE('',*,*,#7531,.F.);
#10120=ORIENTED_EDGE('',*,*,#7532,.F.);
#10121=ORIENTED_EDGE('',*,*,#7533,.T.);
#10122=ORIENTED_EDGE('',*,*,#7534,.T.);
#10123=ORIENTED_EDGE('',*,*,#7531,.T.);
#10124=ORIENTED_EDGE('',*,*,#7535,.T.);
#10125=ORIENTED_EDGE('',*,*,#7536,.F.);
#10126=ORIENTED_EDGE('',*,*,#7537,.F.);
#10127=ORIENTED_EDGE('',*,*,#7538,.F.);
#10128=ORIENTED_EDGE('',*,*,#7539,.T.);
#10129=ORIENTED_EDGE('',*,*,#7540,.T.);
#10130=ORIENTED_EDGE('',*,*,#7537,.T.);
#10131=ORIENTED_EDGE('',*,*,#7541,.T.);
#10132=ORIENTED_EDGE('',*,*,#7542,.T.);
#10133=ORIENTED_EDGE('',*,*,#7543,.T.);
#10134=ORIENTED_EDGE('',*,*,#7538,.T.);
#10135=ORIENTED_EDGE('',*,*,#7544,.T.);
#10136=ORIENTED_EDGE('',*,*,#7545,.T.);
#10137=ORIENTED_EDGE('',*,*,#7536,.T.);
#10138=ORIENTED_EDGE('',*,*,#7546,.T.);
#10139=ORIENTED_EDGE('',*,*,#7532,.T.);
#10140=ORIENTED_EDGE('',*,*,#7547,.T.);
#10141=ORIENTED_EDGE('',*,*,#7548,.T.);
#10142=ORIENTED_EDGE('',*,*,#7549,.T.);
#10143=ORIENTED_EDGE('',*,*,#7530,.T.);
#10144=ORIENTED_EDGE('',*,*,#7550,.T.);
#10145=ORIENTED_EDGE('',*,*,#7551,.T.);
#10146=ORIENTED_EDGE('',*,*,#7541,.F.);
#10147=ORIENTED_EDGE('',*,*,#7547,.F.);
#10148=ORIENTED_EDGE('',*,*,#7534,.F.);
#10149=ORIENTED_EDGE('',*,*,#7552,.F.);
#10150=ORIENTED_EDGE('',*,*,#7535,.F.);
#10151=ORIENTED_EDGE('',*,*,#7549,.F.);
#10152=ORIENTED_EDGE('',*,*,#7553,.F.);
#10153=ORIENTED_EDGE('',*,*,#7554,.F.);
#10154=ORIENTED_EDGE('',*,*,#7548,.F.);
#10155=ORIENTED_EDGE('',*,*,#7555,.T.);
#10156=ORIENTED_EDGE('',*,*,#7556,.T.);
#10157=ORIENTED_EDGE('',*,*,#7557,.F.);
#10158=ORIENTED_EDGE('',*,*,#7553,.T.);
#10159=ORIENTED_EDGE('',*,*,#7420,.F.);
#10160=ORIENTED_EDGE('',*,*,#7558,.T.);
#10161=ORIENTED_EDGE('',*,*,#7559,.T.);
#10162=ORIENTED_EDGE('',*,*,#7560,.T.);
#10163=ORIENTED_EDGE('',*,*,#7561,.T.);
#10164=ORIENTED_EDGE('',*,*,#7425,.F.);
#10165=ORIENTED_EDGE('',*,*,#7426,.F.);
#10166=ORIENTED_EDGE('',*,*,#7561,.F.);
#10167=ORIENTED_EDGE('',*,*,#7562,.F.);
#10168=ORIENTED_EDGE('',*,*,#7563,.F.);
#10169=ORIENTED_EDGE('',*,*,#7560,.F.);
#10170=ORIENTED_EDGE('',*,*,#7564,.T.);
#10171=ORIENTED_EDGE('',*,*,#7565,.T.);
#10172=ORIENTED_EDGE('',*,*,#7566,.F.);
#10173=ORIENTED_EDGE('',*,*,#7562,.T.);
#10174=ORIENTED_EDGE('',*,*,#7567,.T.);
#10175=ORIENTED_EDGE('',*,*,#7568,.T.);
#10176=ORIENTED_EDGE('',*,*,#7569,.T.);
#10177=ORIENTED_EDGE('',*,*,#7570,.T.);
#10178=ORIENTED_EDGE('',*,*,#7571,.T.);
#10179=ORIENTED_EDGE('',*,*,#7572,.T.);
#10180=ORIENTED_EDGE('',*,*,#7573,.T.);
#10181=ORIENTED_EDGE('',*,*,#7570,.F.);
#10182=ORIENTED_EDGE('',*,*,#7567,.F.);
#10183=ORIENTED_EDGE('',*,*,#7574,.T.);
#10184=ORIENTED_EDGE('',*,*,#7575,.T.);
#10185=ORIENTED_EDGE('',*,*,#7576,.F.);
#10186=ORIENTED_EDGE('',*,*,#7573,.F.);
#10187=ORIENTED_EDGE('',*,*,#7577,.T.);
#10188=ORIENTED_EDGE('',*,*,#7578,.T.);
#10189=ORIENTED_EDGE('',*,*,#7574,.F.);
#10190=ORIENTED_EDGE('',*,*,#7579,.T.);
#10191=ORIENTED_EDGE('',*,*,#7568,.F.);
#10192=ORIENTED_EDGE('',*,*,#7580,.T.);
#10193=ORIENTED_EDGE('',*,*,#7581,.T.);
#10194=ORIENTED_EDGE('',*,*,#7582,.T.);
#10195=ORIENTED_EDGE('',*,*,#7572,.F.);
#10196=ORIENTED_EDGE('',*,*,#7583,.T.);
#10197=ORIENTED_EDGE('',*,*,#7581,.F.);
#10198=ORIENTED_EDGE('',*,*,#7584,.F.);
#10199=ORIENTED_EDGE('',*,*,#7585,.F.);
#10200=ORIENTED_EDGE('',*,*,#7586,.F.);
#10201=ORIENTED_EDGE('',*,*,#7587,.F.);
#10202=ORIENTED_EDGE('',*,*,#7588,.F.);
#10203=ORIENTED_EDGE('',*,*,#7528,.F.);
#10204=ORIENTED_EDGE('',*,*,#7589,.F.);
#10205=ORIENTED_EDGE('',*,*,#7590,.F.);
#10206=ORIENTED_EDGE('',*,*,#7591,.F.);
#10207=ORIENTED_EDGE('',*,*,#7556,.F.);
#10208=ORIENTED_EDGE('',*,*,#7592,.F.);
#10209=ORIENTED_EDGE('',*,*,#7593,.F.);
#10210=ORIENTED_EDGE('',*,*,#7594,.F.);
#10211=ORIENTED_EDGE('',*,*,#7565,.F.);
#10212=ORIENTED_EDGE('',*,*,#7595,.F.);
#10213=ORIENTED_EDGE('',*,*,#7596,.F.);
#10214=ORIENTED_EDGE('',*,*,#7597,.F.);
#10215=ORIENTED_EDGE('',*,*,#7598,.F.);
#10216=ORIENTED_EDGE('',*,*,#7599,.F.);
#10217=ORIENTED_EDGE('',*,*,#7600,.F.);
#10218=ORIENTED_EDGE('',*,*,#7579,.F.);
#10219=ORIENTED_EDGE('',*,*,#7583,.F.);
#10220=ORIENTED_EDGE('',*,*,#7571,.F.);
#10221=ORIENTED_EDGE('',*,*,#7569,.F.);
#10222=ORIENTED_EDGE('',*,*,#7601,.T.);
#10223=ORIENTED_EDGE('',*,*,#7584,.T.);
#10224=ORIENTED_EDGE('',*,*,#7602,.T.);
#10225=ORIENTED_EDGE('',*,*,#7603,.T.);
#10226=ORIENTED_EDGE('',*,*,#7604,.T.);
#10227=ORIENTED_EDGE('',*,*,#7605,.T.);
#10228=ORIENTED_EDGE('',*,*,#7601,.F.);
#10229=ORIENTED_EDGE('',*,*,#7606,.T.);
#10230=ORIENTED_EDGE('',*,*,#7607,.T.);
#10231=ORIENTED_EDGE('',*,*,#7608,.T.);
#10232=ORIENTED_EDGE('',*,*,#7604,.F.);
#10233=ORIENTED_EDGE('',*,*,#7609,.T.);
#10234=ORIENTED_EDGE('',*,*,#7610,.T.);
#10235=ORIENTED_EDGE('',*,*,#7611,.T.);
#10236=ORIENTED_EDGE('',*,*,#7607,.F.);
#10237=ORIENTED_EDGE('',*,*,#7612,.T.);
#10238=ORIENTED_EDGE('',*,*,#7613,.T.);
#10239=ORIENTED_EDGE('',*,*,#7614,.T.);
#10240=ORIENTED_EDGE('',*,*,#7610,.F.);
#10241=ORIENTED_EDGE('',*,*,#7615,.T.);
#10242=ORIENTED_EDGE('',*,*,#7616,.T.);
#10243=ORIENTED_EDGE('',*,*,#7617,.T.);
#10244=ORIENTED_EDGE('',*,*,#7613,.F.);
#10245=ORIENTED_EDGE('',*,*,#7618,.T.);
#10246=ORIENTED_EDGE('',*,*,#7619,.T.);
#10247=ORIENTED_EDGE('',*,*,#7620,.T.);
#10248=ORIENTED_EDGE('',*,*,#7616,.F.);
#10249=ORIENTED_EDGE('',*,*,#7621,.T.);
#10250=ORIENTED_EDGE('',*,*,#7602,.F.);
#10251=ORIENTED_EDGE('',*,*,#7622,.T.);
#10252=ORIENTED_EDGE('',*,*,#7619,.F.);
#10253=ORIENTED_EDGE('',*,*,#7623,.T.);
#10254=ORIENTED_EDGE('',*,*,#7617,.F.);
#10255=ORIENTED_EDGE('',*,*,#7624,.T.);
#10256=ORIENTED_EDGE('',*,*,#7625,.F.);
#10257=ORIENTED_EDGE('',*,*,#7626,.T.);
#10258=ORIENTED_EDGE('',*,*,#7620,.F.);
#10259=ORIENTED_EDGE('',*,*,#7627,.F.);
#10260=ORIENTED_EDGE('',*,*,#7628,.F.);
#10261=ORIENTED_EDGE('',*,*,#7624,.F.);
#10262=ORIENTED_EDGE('',*,*,#7629,.F.);
#10263=ORIENTED_EDGE('',*,*,#7622,.F.);
#10264=ORIENTED_EDGE('',*,*,#7600,.T.);
#10265=ORIENTED_EDGE('',*,*,#7630,.F.);
#10266=ORIENTED_EDGE('',*,*,#7631,.F.);
#10267=ORIENTED_EDGE('',*,*,#7632,.F.);
#10268=ORIENTED_EDGE('',*,*,#7598,.T.);
#10269=ORIENTED_EDGE('',*,*,#7633,.F.);
#10270=ORIENTED_EDGE('',*,*,#7627,.T.);
#10271=ORIENTED_EDGE('',*,*,#7603,.F.);
#10272=ORIENTED_EDGE('',*,*,#7623,.F.);
#10273=ORIENTED_EDGE('',*,*,#7621,.F.);
#10274=ORIENTED_EDGE('',*,*,#7618,.F.);
#10275=ORIENTED_EDGE('',*,*,#7615,.F.);
#10276=ORIENTED_EDGE('',*,*,#7612,.F.);
#10277=ORIENTED_EDGE('',*,*,#7609,.F.);
#10278=ORIENTED_EDGE('',*,*,#7606,.F.);
#10279=ORIENTED_EDGE('',*,*,#7634,.T.);
#10280=ORIENTED_EDGE('',*,*,#7566,.T.);
#10281=ORIENTED_EDGE('',*,*,#7594,.T.);
#10282=ORIENTED_EDGE('',*,*,#7635,.T.);
#10283=ORIENTED_EDGE('',*,*,#7591,.T.);
#10284=ORIENTED_EDGE('',*,*,#7636,.T.);
#10285=ORIENTED_EDGE('',*,*,#7637,.T.);
#10286=ORIENTED_EDGE('',*,*,#7557,.T.);
#10287=ORIENTED_EDGE('',*,*,#7517,.F.);
#10288=ORIENTED_EDGE('',*,*,#7638,.T.);
#10289=ORIENTED_EDGE('',*,*,#7636,.F.);
#10290=ORIENTED_EDGE('',*,*,#7590,.T.);
#10291=ORIENTED_EDGE('',*,*,#7639,.T.);
#10292=ORIENTED_EDGE('',*,*,#7588,.T.);
#10293=ORIENTED_EDGE('',*,*,#7640,.T.);
#10294=ORIENTED_EDGE('',*,*,#7641,.T.);
#10295=ORIENTED_EDGE('',*,*,#7529,.T.);
#10296=ORIENTED_EDGE('',*,*,#7640,.F.);
#10297=ORIENTED_EDGE('',*,*,#7642,.T.);
#10298=ORIENTED_EDGE('',*,*,#7643,.T.);
#10299=ORIENTED_EDGE('',*,*,#7644,.T.);
#10300=ORIENTED_EDGE('',*,*,#7645,.T.);
#10301=ORIENTED_EDGE('',*,*,#7646,.T.);
#10302=ORIENTED_EDGE('',*,*,#7643,.F.);
#10303=ORIENTED_EDGE('',*,*,#7647,.T.);
#10304=ORIENTED_EDGE('',*,*,#7645,.F.);
#10305=ORIENTED_EDGE('',*,*,#7648,.T.);
#10306=ORIENTED_EDGE('',*,*,#7649,.T.);
#10307=ORIENTED_EDGE('',*,*,#7650,.T.);
#10308=ORIENTED_EDGE('',*,*,#7651,.T.);
#10309=ORIENTED_EDGE('',*,*,#7652,.T.);
#10310=ORIENTED_EDGE('',*,*,#7649,.F.);
#10311=ORIENTED_EDGE('',*,*,#7653,.T.);
#10312=ORIENTED_EDGE('',*,*,#7651,.F.);
#10313=ORIENTED_EDGE('',*,*,#7625,.T.);
#10314=ORIENTED_EDGE('',*,*,#7654,.T.);
#10315=ORIENTED_EDGE('',*,*,#7655,.T.);
#10316=ORIENTED_EDGE('',*,*,#7656,.T.);
#10317=ORIENTED_EDGE('',*,*,#7657,.T.);
#10318=ORIENTED_EDGE('',*,*,#7654,.F.);
#10319=ORIENTED_EDGE('',*,*,#7628,.T.);
#10320=ORIENTED_EDGE('',*,*,#7656,.F.);
#10321=ORIENTED_EDGE('',*,*,#7633,.T.);
#10322=ORIENTED_EDGE('',*,*,#7658,.T.);
#10323=ORIENTED_EDGE('',*,*,#7659,.T.);
#10324=ORIENTED_EDGE('',*,*,#7660,.T.);
#10325=ORIENTED_EDGE('',*,*,#7658,.F.);
#10326=ORIENTED_EDGE('',*,*,#7597,.T.);
#10327=ORIENTED_EDGE('',*,*,#7661,.T.);
#10328=ORIENTED_EDGE('',*,*,#7416,.F.);
#10329=ORIENTED_EDGE('',*,*,#7422,.T.);
#10330=ORIENTED_EDGE('',*,*,#7661,.F.);
#10331=ORIENTED_EDGE('',*,*,#7596,.T.);
#10332=ORIENTED_EDGE('',*,*,#7662,.T.);
#10333=ORIENTED_EDGE('',*,*,#7514,.F.);
#10334=ORIENTED_EDGE('',*,*,#7639,.F.);
#10335=ORIENTED_EDGE('',*,*,#7589,.T.);
#10336=ORIENTED_EDGE('',*,*,#7527,.F.);
#10337=ORIENTED_EDGE('',*,*,#7523,.F.);
#10338=ORIENTED_EDGE('',*,*,#7663,.T.);
#10339=ORIENTED_EDGE('',*,*,#7413,.F.);
#10340=ORIENTED_EDGE('',*,*,#7662,.F.);
#10341=ORIENTED_EDGE('',*,*,#7595,.T.);
#10342=ORIENTED_EDGE('',*,*,#7564,.F.);
#10343=ORIENTED_EDGE('',*,*,#7559,.F.);
#10344=ORIENTED_EDGE('',*,*,#7664,.T.);
#10345=ORIENTED_EDGE('',*,*,#7545,.F.);
#10346=ORIENTED_EDGE('',*,*,#7665,.T.);
#10347=ORIENTED_EDGE('',*,*,#7635,.F.);
#10348=ORIENTED_EDGE('',*,*,#7593,.T.);
#10349=ORIENTED_EDGE('',*,*,#7666,.T.);
#10350=ORIENTED_EDGE('',*,*,#7542,.F.);
#10351=ORIENTED_EDGE('',*,*,#7666,.F.);
#10352=ORIENTED_EDGE('',*,*,#7592,.T.);
#10353=ORIENTED_EDGE('',*,*,#7555,.F.);
#10354=ORIENTED_EDGE('',*,*,#7551,.F.);
#10355=ORIENTED_EDGE('',*,*,#7667,.T.);
#10356=ORIENTED_EDGE('',*,*,#7614,.F.);
#10357=ORIENTED_EDGE('',*,*,#7626,.F.);
#10358=ORIENTED_EDGE('',*,*,#7653,.F.);
#10359=ORIENTED_EDGE('',*,*,#7668,.F.);
#10360=ORIENTED_EDGE('',*,*,#7611,.F.);
#10361=ORIENTED_EDGE('',*,*,#7668,.T.);
#10362=ORIENTED_EDGE('',*,*,#7648,.F.);
#10363=ORIENTED_EDGE('',*,*,#7669,.T.);
#10364=ORIENTED_EDGE('',*,*,#7608,.F.);
#10365=ORIENTED_EDGE('',*,*,#7669,.F.);
#10366=ORIENTED_EDGE('',*,*,#7647,.F.);
#10367=ORIENTED_EDGE('',*,*,#7670,.F.);
#10368=ORIENTED_EDGE('',*,*,#7605,.F.);
#10369=ORIENTED_EDGE('',*,*,#7670,.T.);
#10370=ORIENTED_EDGE('',*,*,#7642,.F.);
#10371=ORIENTED_EDGE('',*,*,#7587,.T.);
#10372=ORIENTED_EDGE('',*,*,#7671,.F.);
#10373=ORIENTED_EDGE('',*,*,#7672,.F.);
#10374=ORIENTED_EDGE('',*,*,#7673,.F.);
#10375=ORIENTED_EDGE('',*,*,#7585,.T.);
#10376=ORIENTED_EDGE('',*,*,#7540,.F.);
#10377=ORIENTED_EDGE('',*,*,#7674,.F.);
#10378=ORIENTED_EDGE('',*,*,#7665,.F.);
#10379=ORIENTED_EDGE('',*,*,#7544,.F.);
#10380=ORIENTED_EDGE('',*,*,#7543,.F.);
#10381=ORIENTED_EDGE('',*,*,#7667,.F.);
#10382=ORIENTED_EDGE('',*,*,#7550,.F.);
#10383=ORIENTED_EDGE('',*,*,#7546,.F.);
#10384=ORIENTED_EDGE('',*,*,#7634,.F.);
#10385=ORIENTED_EDGE('',*,*,#7674,.T.);
#10386=ORIENTED_EDGE('',*,*,#7539,.F.);
#10387=ORIENTED_EDGE('',*,*,#7552,.T.);
#10388=ORIENTED_EDGE('',*,*,#7533,.F.);
#10389=ORIENTED_EDGE('',*,*,#7554,.T.);
#10390=ORIENTED_EDGE('',*,*,#7637,.F.);
#10391=ORIENTED_EDGE('',*,*,#7675,.T.);
#10392=ORIENTED_EDGE('',*,*,#7511,.F.);
#10393=ORIENTED_EDGE('',*,*,#7524,.T.);
#10394=ORIENTED_EDGE('',*,*,#7505,.F.);
#10395=ORIENTED_EDGE('',*,*,#7526,.T.);
#10396=ORIENTED_EDGE('',*,*,#7641,.F.);
#10397=ORIENTED_EDGE('',*,*,#7644,.F.);
#10398=ORIENTED_EDGE('',*,*,#7646,.F.);
#10399=ORIENTED_EDGE('',*,*,#7650,.F.);
#10400=ORIENTED_EDGE('',*,*,#7652,.F.);
#10401=ORIENTED_EDGE('',*,*,#7655,.F.);
#10402=ORIENTED_EDGE('',*,*,#7657,.F.);
#10403=ORIENTED_EDGE('',*,*,#7659,.F.);
#10404=ORIENTED_EDGE('',*,*,#7660,.F.);
#10405=ORIENTED_EDGE('',*,*,#7421,.T.);
#10406=ORIENTED_EDGE('',*,*,#7410,.F.);
#10407=ORIENTED_EDGE('',*,*,#7424,.T.);
#10408=ORIENTED_EDGE('',*,*,#7427,.F.);
#10409=ORIENTED_EDGE('',*,*,#7563,.T.);
#10410=ORIENTED_EDGE('',*,*,#7405,.T.);
#10411=ORIENTED_EDGE('',*,*,#7390,.F.);
#10412=ORIENTED_EDGE('',*,*,#7439,.T.);
#10413=ORIENTED_EDGE('',*,*,#7397,.F.);
#10414=ORIENTED_EDGE('',*,*,#7402,.T.);
#10415=ORIENTED_EDGE('',*,*,#7472,.F.);
#10416=ORIENTED_EDGE('',*,*,#7501,.T.);
#10417=ORIENTED_EDGE('',*,*,#7477,.F.);
#10418=ORIENTED_EDGE('',*,*,#7371,.T.);
#10419=ORIENTED_EDGE('',*,*,#7381,.F.);
#10420=ORIENTED_EDGE('',*,*,#7383,.T.);
#10421=ORIENTED_EDGE('',*,*,#7376,.F.);
#10422=ORIENTED_EDGE('',*,*,#7374,.T.);
#10423=ORIENTED_EDGE('',*,*,#7359,.F.);
#10424=ORIENTED_EDGE('',*,*,#7433,.T.);
#10425=ORIENTED_EDGE('',*,*,#7366,.F.);
#10426=ORIENTED_EDGE('',*,*,#7512,.F.);
#10427=ORIENTED_EDGE('',*,*,#7675,.F.);
#10428=ORIENTED_EDGE('',*,*,#7638,.F.);
#10429=ORIENTED_EDGE('',*,*,#7516,.F.);
#10430=ORIENTED_EDGE('',*,*,#7515,.F.);
#10431=ORIENTED_EDGE('',*,*,#7663,.F.);
#10432=ORIENTED_EDGE('',*,*,#7522,.F.);
#10433=ORIENTED_EDGE('',*,*,#7518,.F.);
#10434=ORIENTED_EDGE('',*,*,#7676,.T.);
#10435=ORIENTED_EDGE('',*,*,#7631,.T.);
#10436=ORIENTED_EDGE('',*,*,#7677,.T.);
#10437=ORIENTED_EDGE('',*,*,#7678,.T.);
#10438=ORIENTED_EDGE('',*,*,#7679,.T.);
#10439=ORIENTED_EDGE('',*,*,#7680,.T.);
#10440=ORIENTED_EDGE('',*,*,#7681,.T.);
#10441=ORIENTED_EDGE('',*,*,#7682,.T.);
#10442=ORIENTED_EDGE('',*,*,#7599,.T.);
#10443=ORIENTED_EDGE('',*,*,#7679,.F.);
#10444=ORIENTED_EDGE('',*,*,#7632,.T.);
#10445=ORIENTED_EDGE('',*,*,#7676,.F.);
#10446=ORIENTED_EDGE('',*,*,#7683,.T.);
#10447=ORIENTED_EDGE('',*,*,#7677,.F.);
#10448=ORIENTED_EDGE('',*,*,#7630,.T.);
#10449=ORIENTED_EDGE('',*,*,#7682,.F.);
#10450=ORIENTED_EDGE('',*,*,#7684,.T.);
#10451=ORIENTED_EDGE('',*,*,#7680,.F.);
#10452=ORIENTED_EDGE('',*,*,#7683,.F.);
#10453=ORIENTED_EDGE('',*,*,#7678,.F.);
#10454=ORIENTED_EDGE('',*,*,#7684,.F.);
#10455=ORIENTED_EDGE('',*,*,#7681,.F.);
#10456=ORIENTED_EDGE('',*,*,#7685,.T.);
#10457=ORIENTED_EDGE('',*,*,#7686,.T.);
#10458=ORIENTED_EDGE('',*,*,#7685,.F.);
#10459=ORIENTED_EDGE('',*,*,#7687,.T.);
#10460=ORIENTED_EDGE('',*,*,#7672,.T.);
#10461=ORIENTED_EDGE('',*,*,#7688,.T.);
#10462=ORIENTED_EDGE('',*,*,#7689,.T.);
#10463=ORIENTED_EDGE('',*,*,#7690,.T.);
#10464=ORIENTED_EDGE('',*,*,#7691,.T.);
#10465=ORIENTED_EDGE('',*,*,#7692,.T.);
#10466=ORIENTED_EDGE('',*,*,#7693,.T.);
#10467=ORIENTED_EDGE('',*,*,#7586,.T.);
#10468=ORIENTED_EDGE('',*,*,#7691,.F.);
#10469=ORIENTED_EDGE('',*,*,#7673,.T.);
#10470=ORIENTED_EDGE('',*,*,#7687,.F.);
#10471=ORIENTED_EDGE('',*,*,#7694,.T.);
#10472=ORIENTED_EDGE('',*,*,#7688,.F.);
#10473=ORIENTED_EDGE('',*,*,#7671,.T.);
#10474=ORIENTED_EDGE('',*,*,#7693,.F.);
#10475=ORIENTED_EDGE('',*,*,#7695,.T.);
#10476=ORIENTED_EDGE('',*,*,#7692,.F.);
#10477=ORIENTED_EDGE('',*,*,#7694,.F.);
#10478=ORIENTED_EDGE('',*,*,#7690,.F.);
#10479=ORIENTED_EDGE('',*,*,#7696,.T.);
#10480=ORIENTED_EDGE('',*,*,#7697,.T.);
#10481=ORIENTED_EDGE('',*,*,#7696,.F.);
#10482=ORIENTED_EDGE('',*,*,#7689,.F.);
#10483=ORIENTED_EDGE('',*,*,#7695,.F.);
#10484=ORIENTED_EDGE('',*,*,#7629,.T.);
#10485=ORIENTED_EDGE('',*,*,#7698,.T.);
#10486=ORIENTED_EDGE('',*,*,#7699,.T.);
#10487=ORIENTED_EDGE('',*,*,#7698,.F.);
#10488=ORIENTED_EDGE('',*,*,#7699,.F.);
#10489=ORIENTED_EDGE('',*,*,#7700,.T.);
#10490=ORIENTED_EDGE('',*,*,#7701,.F.);
#10491=ORIENTED_EDGE('',*,*,#7700,.F.);
#10492=ORIENTED_EDGE('',*,*,#7702,.T.);
#10493=ORIENTED_EDGE('',*,*,#7703,.T.);
#10494=ORIENTED_EDGE('',*,*,#7701,.T.);
#10495=ORIENTED_EDGE('',*,*,#7703,.F.);
#10496=ORIENTED_EDGE('',*,*,#7580,.F.);
#10497=ORIENTED_EDGE('',*,*,#7576,.T.);
#10498=ORIENTED_EDGE('',*,*,#7704,.T.);
#10499=ORIENTED_EDGE('',*,*,#7705,.F.);
#10500=ORIENTED_EDGE('',*,*,#7702,.F.);
#10501=ORIENTED_EDGE('',*,*,#7697,.F.);
#10502=ORIENTED_EDGE('',*,*,#7686,.F.);
#10503=ORIENTED_EDGE('',*,*,#7490,.F.);
#10504=ORIENTED_EDGE('',*,*,#7706,.T.);
#10505=ORIENTED_EDGE('',*,*,#7468,.T.);
#10506=ORIENTED_EDGE('',*,*,#7500,.F.);
#10507=ORIENTED_EDGE('',*,*,#7495,.F.);
#10508=ORIENTED_EDGE('',*,*,#7707,.T.);
#10509=ORIENTED_EDGE('',*,*,#7469,.T.);
#10510=ORIENTED_EDGE('',*,*,#7706,.F.);
#10511=ORIENTED_EDGE('',*,*,#7481,.F.);
#10512=ORIENTED_EDGE('',*,*,#7498,.T.);
#10513=ORIENTED_EDGE('',*,*,#7470,.T.);
#10514=ORIENTED_EDGE('',*,*,#7707,.F.);
#10515=ORIENTED_EDGE('',*,*,#7456,.F.);
#10516=ORIENTED_EDGE('',*,*,#7708,.T.);
#10517=ORIENTED_EDGE('',*,*,#7444,.T.);
#10518=ORIENTED_EDGE('',*,*,#7463,.F.);
#10519=ORIENTED_EDGE('',*,*,#7459,.F.);
#10520=ORIENTED_EDGE('',*,*,#7709,.T.);
#10521=ORIENTED_EDGE('',*,*,#7445,.T.);
#10522=ORIENTED_EDGE('',*,*,#7708,.F.);
#10523=ORIENTED_EDGE('',*,*,#7449,.F.);
#10524=ORIENTED_EDGE('',*,*,#7461,.T.);
#10525=ORIENTED_EDGE('',*,*,#7446,.T.);
#10526=ORIENTED_EDGE('',*,*,#7709,.F.);
#10527=ORIENTED_EDGE('',*,*,#7582,.F.);
#10528=ORIENTED_EDGE('',*,*,#7705,.T.);
#10529=ORIENTED_EDGE('',*,*,#7710,.T.);
#10530=ORIENTED_EDGE('',*,*,#7577,.F.);
#10531=ORIENTED_EDGE('',*,*,#7710,.F.);
#10532=ORIENTED_EDGE('',*,*,#7704,.F.);
#10533=ORIENTED_EDGE('',*,*,#7575,.F.);
#10534=ORIENTED_EDGE('',*,*,#7578,.F.);
#10535=ORIENTED_EDGE('',*,*,#7414,.F.);
#10536=ORIENTED_EDGE('',*,*,#7664,.F.);
#10537=ORIENTED_EDGE('',*,*,#7558,.F.);
#10538=ORIENTED_EDGE('',*,*,#7419,.F.);
#13546=PLANE('',#15138);
#13547=PLANE('',#15142);
#13548=PLANE('',#15143);
#13549=PLANE('',#15146);
#13550=PLANE('',#15147);
#13551=PLANE('',#15150);
#13552=PLANE('',#15151);
#13553=PLANE('',#15152);
#13554=PLANE('',#15156);
#13555=PLANE('',#15157);
#13556=PLANE('',#15160);
#13557=PLANE('',#15161);
#13558=PLANE('',#15162);
#13559=PLANE('',#15163);
#13560=PLANE('',#15164);
#13561=PLANE('',#15165);
#13562=PLANE('',#15166);
#13563=PLANE('',#15167);
#13564=PLANE('',#15173);
#13565=PLANE('',#15179);
#13566=PLANE('',#15182);
#13567=PLANE('',#15183);
#13568=PLANE('',#15184);
#13569=PLANE('',#15185);
#13570=PLANE('',#15186);
#13571=PLANE('',#15187);
#13572=PLANE('',#15188);
#13573=PLANE('',#15189);
#13574=PLANE('',#15190);
#13575=PLANE('',#15191);
#13576=PLANE('',#15194);
#13577=PLANE('',#15195);
#13578=PLANE('',#15198);
#13579=PLANE('',#15199);
#13580=PLANE('',#15200);
#13581=PLANE('',#15201);
#13582=PLANE('',#15202);
#13583=PLANE('',#15203);
#13584=PLANE('',#15204);
#13585=PLANE('',#15205);
#13586=PLANE('',#15206);
#13587=PLANE('',#15207);
#13588=PLANE('',#15208);
#13589=PLANE('',#15209);
#13590=PLANE('',#15210);
#13591=PLANE('',#15211);
#13592=PLANE('',#15212);
#13593=PLANE('',#15213);
#13594=PLANE('',#15214);
#13595=PLANE('',#15215);
#13596=PLANE('',#15216);
#13597=PLANE('',#15217);
#13598=PLANE('',#15218);
#13599=PLANE('',#15219);
#13600=PLANE('',#15220);
#13601=PLANE('',#15221);
#13602=PLANE('',#15222);
#13603=PLANE('',#15223);
#13604=PLANE('',#15224);
#13605=PLANE('',#15225);
#13606=PLANE('',#15226);
#13607=PLANE('',#15227);
#13608=PLANE('',#15228);
#13609=PLANE('',#15229);
#13610=PLANE('',#15230);
#13611=PLANE('',#15231);
#13612=PLANE('',#15232);
#13613=PLANE('',#15233);
#13614=PLANE('',#15234);
#13615=PLANE('',#15235);
#13616=PLANE('',#15236);
#13617=PLANE('',#15237);
#13618=PLANE('',#15238);
#13619=PLANE('',#15241);
#13620=PLANE('',#15245);
#13621=PLANE('',#15249);
#13622=PLANE('',#15253);
#13623=PLANE('',#15259);
#13624=PLANE('',#15263);
#13625=PLANE('',#15264);
#13626=PLANE('',#15265);
#13627=PLANE('',#15266);
#13628=PLANE('',#15267);
#13629=PLANE('',#15271);
#13630=PLANE('',#15275);
#13631=PLANE('',#15278);
#13632=PLANE('',#15281);
#13633=PLANE('',#15282);
#13634=PLANE('',#15283);
#13635=PLANE('',#15284);
#13636=PLANE('',#15285);
#13637=PLANE('',#15286);
#13638=PLANE('',#15287);
#13639=PLANE('',#15289);
#13640=PLANE('',#15291);
#13641=PLANE('',#15292);
#13642=PLANE('',#15293);
#13643=PLANE('',#15294);
#13644=PLANE('',#15295);
#13645=PLANE('',#15311);
#13646=PLANE('',#15312);
#13647=PLANE('',#15313);
#13648=PLANE('',#15314);
#13649=PLANE('',#15315);
#13650=PLANE('',#15316);
#13651=PLANE('',#15317);
#13652=PLANE('',#15318);
#13653=PLANE('',#15319);
#13654=PLANE('',#15320);
#13655=PLANE('',#15321);
#13656=PLANE('',#15322);
#14069=ADVANCED_FACE('',(#1501),#13546,.T.);
#14070=ADVANCED_FACE('',(#1502),#1311,.T.);
#14071=ADVANCED_FACE('',(#1503),#13547,.T.);
#14072=ADVANCED_FACE('',(#1504),#13548,.T.);
#14073=ADVANCED_FACE('',(#1505),#708,.T.);
#14074=ADVANCED_FACE('',(#1506),#13549,.T.);
#14075=ADVANCED_FACE('',(#1507),#13550,.T.);
#14076=ADVANCED_FACE('',(#1508),#1312,.T.);
#14077=ADVANCED_FACE('',(#1509),#13551,.T.);
#14078=ADVANCED_FACE('',(#1510,#654),#13552,.F.);
#14079=ADVANCED_FACE('',(#1511),#13553,.T.);
#14080=ADVANCED_FACE('',(#1512),#1313,.T.);
#14081=ADVANCED_FACE('',(#1513),#13554,.T.);
#14082=ADVANCED_FACE('',(#1514),#13555,.T.);
#14083=ADVANCED_FACE('',(#1515),#709,.T.);
#14084=ADVANCED_FACE('',(#1516),#13556,.T.);
#14085=ADVANCED_FACE('',(#1517),#13557,.T.);
#14086=ADVANCED_FACE('',(#1518),#13558,.T.);
#14087=ADVANCED_FACE('',(#1519),#13559,.T.);
#14088=ADVANCED_FACE('',(#1520),#13560,.T.);
#14089=ADVANCED_FACE('',(#1521),#13561,.T.);
#14090=ADVANCED_FACE('',(#1522),#13562,.T.);
#14091=ADVANCED_FACE('',(#1523),#13563,.T.);
#14092=ADVANCED_FACE('',(#1524),#1314,.F.);
#14093=ADVANCED_FACE('',(#1525),#710,.F.);
#14094=ADVANCED_FACE('',(#1526,#655),#13564,.T.);
#14095=ADVANCED_FACE('',(#1527),#1315,.F.);
#14096=ADVANCED_FACE('',(#1528),#711,.F.);
#14097=ADVANCED_FACE('',(#1529,#656),#13565,.F.);
#14098=ADVANCED_FACE('',(#1530),#1316,.F.);
#14099=ADVANCED_FACE('',(#1531,#657),#13566,.F.);
#14100=ADVANCED_FACE('',(#1532),#13567,.T.);
#14101=ADVANCED_FACE('',(#1533),#13568,.T.);
#14102=ADVANCED_FACE('',(#1534),#13569,.T.);
#14103=ADVANCED_FACE('',(#1535),#13570,.T.);
#14104=ADVANCED_FACE('',(#1536),#13571,.T.);
#14105=ADVANCED_FACE('',(#1537),#13572,.T.);
#14106=ADVANCED_FACE('',(#1538),#13573,.F.);
#14107=ADVANCED_FACE('',(#1539),#13574,.F.);
#14108=ADVANCED_FACE('',(#1540),#13575,.F.);
#14109=ADVANCED_FACE('',(#1541),#1317,.F.);
#14110=ADVANCED_FACE('',(#1542,#658),#13576,.F.);
#14111=ADVANCED_FACE('',(#1543),#13577,.T.);
#14112=ADVANCED_FACE('',(#1544),#1318,.T.);
#14113=ADVANCED_FACE('',(#1545),#13578,.T.);
#14114=ADVANCED_FACE('',(#1546),#13579,.T.);
#14115=ADVANCED_FACE('',(#1547),#13580,.T.);
#14116=ADVANCED_FACE('',(#1548),#13581,.T.);
#14117=ADVANCED_FACE('',(#1549),#13582,.T.);
#14118=ADVANCED_FACE('',(#1550),#13583,.T.);
#14119=ADVANCED_FACE('',(#1551),#13584,.T.);
#14120=ADVANCED_FACE('',(#1552),#13585,.F.);
#14121=ADVANCED_FACE('',(#1553),#13586,.F.);
#14122=ADVANCED_FACE('',(#1554),#13587,.F.);
#14123=ADVANCED_FACE('',(#1555,#659),#13588,.T.);
#14124=ADVANCED_FACE('',(#1556),#13589,.T.);
#14125=ADVANCED_FACE('',(#1557),#13590,.T.);
#14126=ADVANCED_FACE('',(#1558),#13591,.T.);
#14127=ADVANCED_FACE('',(#1559),#13592,.T.);
#14128=ADVANCED_FACE('',(#1560),#13593,.T.);
#14129=ADVANCED_FACE('',(#1561),#13594,.T.);
#14130=ADVANCED_FACE('',(#1562),#13595,.T.);
#14131=ADVANCED_FACE('',(#1563),#13596,.T.);
#14132=ADVANCED_FACE('',(#1564),#13597,.T.);
#14133=ADVANCED_FACE('',(#1565),#13598,.T.);
#14134=ADVANCED_FACE('',(#1566),#13599,.T.);
#14135=ADVANCED_FACE('',(#1567),#13600,.T.);
#14136=ADVANCED_FACE('',(#1568),#13601,.T.);
#14137=ADVANCED_FACE('',(#1569),#13602,.T.);
#14138=ADVANCED_FACE('',(#1570),#13603,.T.);
#14139=ADVANCED_FACE('',(#1571),#13604,.T.);
#14140=ADVANCED_FACE('',(#1572),#13605,.T.);
#14141=ADVANCED_FACE('',(#1573),#13606,.T.);
#14142=ADVANCED_FACE('',(#1574),#13607,.T.);
#14143=ADVANCED_FACE('',(#1575),#13608,.T.);
#14144=ADVANCED_FACE('',(#1576),#13609,.T.);
#14145=ADVANCED_FACE('',(#1577),#13610,.T.);
#14146=ADVANCED_FACE('',(#1578),#13611,.T.);
#14147=ADVANCED_FACE('',(#1579),#13612,.T.);
#14148=ADVANCED_FACE('',(#1580),#13613,.T.);
#14149=ADVANCED_FACE('',(#1581),#13614,.F.);
#14150=ADVANCED_FACE('',(#1582),#13615,.F.);
#14151=ADVANCED_FACE('',(#1583),#13616,.T.);
#14152=ADVANCED_FACE('',(#1584),#13617,.T.);
#14153=ADVANCED_FACE('',(#1585,#660),#13618,.T.);
#14154=ADVANCED_FACE('',(#1586),#13619,.T.);
#14155=ADVANCED_FACE('',(#1587),#1319,.T.);
#14156=ADVANCED_FACE('',(#1588),#13620,.T.);
#14157=ADVANCED_FACE('',(#1589),#1320,.T.);
#14158=ADVANCED_FACE('',(#1590),#13621,.T.);
#14159=ADVANCED_FACE('',(#1591),#1321,.T.);
#14160=ADVANCED_FACE('',(#1592),#13622,.T.);
#14161=ADVANCED_FACE('',(#1593),#1322,.T.);
#14162=ADVANCED_FACE('',(#1594),#712,.T.);
#14163=ADVANCED_FACE('',(#1595,#661),#13623,.T.);
#14164=ADVANCED_FACE('',(#1596),#713,.T.);
#14165=ADVANCED_FACE('',(#1597),#13624,.F.);
#14166=ADVANCED_FACE('',(#1598),#13625,.T.);
#14167=ADVANCED_FACE('',(#1599),#13626,.T.);
#14168=ADVANCED_FACE('',(#1600),#13627,.T.);
#14169=ADVANCED_FACE('',(#1601),#13628,.T.);
#14170=ADVANCED_FACE('',(#1602),#1323,.T.);
#14171=ADVANCED_FACE('',(#1603),#13629,.T.);
#14172=ADVANCED_FACE('',(#1604),#1324,.T.);
#14173=ADVANCED_FACE('',(#1605),#13630,.T.);
#14174=ADVANCED_FACE('',(#1606),#1325,.T.);
#14175=ADVANCED_FACE('',(#1607),#13631,.T.);
#14176=ADVANCED_FACE('',(#1608),#1326,.T.);
#14177=ADVANCED_FACE('',(#1609),#13632,.T.);
#14178=ADVANCED_FACE('',(#1610),#13633,.T.);
#14179=ADVANCED_FACE('',(#1611),#13634,.T.);
#14180=ADVANCED_FACE('',(#1612),#13635,.T.);
#14181=ADVANCED_FACE('',(#1613),#13636,.T.);
#14182=ADVANCED_FACE('',(#1614),#13637,.T.);
#14183=ADVANCED_FACE('',(#1615),#13638,.T.);
#14184=ADVANCED_FACE('',(#1616),#714,.T.);
#14185=ADVANCED_FACE('',(#1617),#13639,.T.);
#14186=ADVANCED_FACE('',(#1618),#715,.T.);
#14187=ADVANCED_FACE('',(#1619),#13640,.T.);
#14188=ADVANCED_FACE('',(#1620),#13641,.T.);
#14189=ADVANCED_FACE('',(#1621,#662,#663),#13642,.T.);
#14190=ADVANCED_FACE('',(#1622),#13643,.T.);
#14191=ADVANCED_FACE('',(#1623),#13644,.T.);
#14192=ADVANCED_FACE('',(#1624),#105,.T.);
#14193=ADVANCED_FACE('',(#1625),#1327,.F.);
#14194=ADVANCED_FACE('',(#1626),#106,.T.);
#14195=ADVANCED_FACE('',(#1627),#107,.T.);
#14196=ADVANCED_FACE('',(#1628),#716,.F.);
#14197=ADVANCED_FACE('',(#1629),#108,.T.);
#14198=ADVANCED_FACE('',(#1630),#1328,.F.);
#14199=ADVANCED_FACE('',(#1631),#109,.T.);
#14200=ADVANCED_FACE('',(#1632),#110,.T.);
#14201=ADVANCED_FACE('',(#1633),#717,.F.);
#14202=ADVANCED_FACE('',(#1634),#1329,.F.);
#14203=ADVANCED_FACE('',(#1635),#718,.F.);
#14204=ADVANCED_FACE('',(#1636),#1330,.F.);
#14205=ADVANCED_FACE('',(#1637,#664),#13645,.F.);
#14206=ADVANCED_FACE('',(#1638),#13646,.T.);
#14207=ADVANCED_FACE('',(#1639),#13647,.T.);
#14208=ADVANCED_FACE('',(#1640),#13648,.F.);
#14209=ADVANCED_FACE('',(#1641),#13649,.F.);
#14210=ADVANCED_FACE('',(#1642),#13650,.F.);
#14211=ADVANCED_FACE('',(#1643),#13651,.F.);
#14212=ADVANCED_FACE('',(#1644),#13652,.F.);
#14213=ADVANCED_FACE('',(#1645),#13653,.F.);
#14214=ADVANCED_FACE('',(#1646),#13654,.F.);
#14215=ADVANCED_FACE('',(#1647),#13655,.F.);
#14216=ADVANCED_FACE('',(#1648),#13656,.T.);
#14778=CLOSED_SHELL('',(#14069,#14070,#14071,#14072,#14073,#14074,#14075,
#14076,#14077,#14078,#14079,#14080,#14081,#14082,#14083,#14084,#14085,#14086,
#14087,#14088,#14089,#14090,#14091,#14092,#14093,#14094,#14095,#14096,#14097,
#14098,#14099,#14100,#14101,#14102,#14103,#14104,#14105,#14106,#14107,#14108,
#14109,#14110,#14111,#14112,#14113,#14114,#14115,#14116,#14117,#14118,#14119,
#14120,#14121,#14122,#14123,#14124,#14125,#14126,#14127,#14128,#14129,#14130,
#14131,#14132,#14133,#14134,#14135,#14136,#14137,#14138,#14139,#14140,#14141,
#14142,#14143,#14144,#14145,#14146,#14147,#14148,#14149,#14150,#14151,#14152,
#14153,#14154,#14155,#14156,#14157,#14158,#14159,#14160,#14161,#14162,#14163,
#14164,#14165,#14166,#14167,#14168,#14169,#14170,#14171,#14172,#14173,#14174,
#14175,#14176,#14177,#14178,#14179,#14180,#14181,#14182,#14183,#14184,#14185,
#14186,#14187,#14188,#14189,#14190,#14191,#14192,#14193,#14194,#14195,#14196,
#14197,#14198,#14199,#14200,#14201,#14202,#14203,#14204,#14205,#14206,#14207,
#14208,#14209,#14210,#14211,#14212,#14213,#14214,#14215,#14216));
#15137=AXIS2_PLACEMENT_3D('',#20523,#16749,#16750);
#15138=AXIS2_PLACEMENT_3D('',#20524,#16751,#16752);
#15139=AXIS2_PLACEMENT_3D('',#20533,#16757,#16758);
#15140=AXIS2_PLACEMENT_3D('',#20537,#16760,#16761);
#15141=AXIS2_PLACEMENT_3D('',#20538,#16762,#16763);
#15142=AXIS2_PLACEMENT_3D('',#20539,#16764,#16765);
#15143=AXIS2_PLACEMENT_3D('',#20545,#16769,#16770);
#15144=AXIS2_PLACEMENT_3D('',#20551,#16774,#16775);
#15145=AXIS2_PLACEMENT_3D('',#20554,#16777,#16778);
#15146=AXIS2_PLACEMENT_3D('',#20555,#16779,#16780);
#15147=AXIS2_PLACEMENT_3D('',#20559,#16783,#16784);
#15148=AXIS2_PLACEMENT_3D('',#20565,#16788,#16789);
#15149=AXIS2_PLACEMENT_3D('',#20568,#16791,#16792);
#15150=AXIS2_PLACEMENT_3D('',#20569,#16793,#16794);
#15151=AXIS2_PLACEMENT_3D('',#20573,#16797,#16798);
#15152=AXIS2_PLACEMENT_3D('',#20587,#16806,#16807);
#15153=AXIS2_PLACEMENT_3D('',#20596,#16812,#16813);
#15154=AXIS2_PLACEMENT_3D('',#20600,#16815,#16816);
#15155=AXIS2_PLACEMENT_3D('',#20601,#16817,#16818);
#15156=AXIS2_PLACEMENT_3D('',#20602,#16819,#16820);
#15157=AXIS2_PLACEMENT_3D('',#20608,#16824,#16825);
#15158=AXIS2_PLACEMENT_3D('',#20614,#16829,#16830);
#15159=AXIS2_PLACEMENT_3D('',#20617,#16832,#16833);
#15160=AXIS2_PLACEMENT_3D('',#20618,#16834,#16835);
#15161=AXIS2_PLACEMENT_3D('',#20622,#16838,#16839);
#15162=AXIS2_PLACEMENT_3D('',#20629,#16843,#16844);
#15163=AXIS2_PLACEMENT_3D('',#20635,#16848,#16849);
#15164=AXIS2_PLACEMENT_3D('',#20643,#16854,#16855);
#15165=AXIS2_PLACEMENT_3D('',#20651,#16860,#16861);
#15166=AXIS2_PLACEMENT_3D('',#20655,#16864,#16865);
#15167=AXIS2_PLACEMENT_3D('',#20659,#16868,#16869);
#15168=AXIS2_PLACEMENT_3D('',#20665,#16873,#16874);
#15169=AXIS2_PLACEMENT_3D('',#20667,#16875,#16876);
#15170=AXIS2_PLACEMENT_3D('',#20670,#16878,#16879);
#15171=AXIS2_PLACEMENT_3D('',#20671,#16880,#16881);
#15172=AXIS2_PLACEMENT_3D('',#20674,#16883,#16884);
#15173=AXIS2_PLACEMENT_3D('',#20675,#16885,#16886);
#15174=AXIS2_PLACEMENT_3D('',#20677,#16888,#16889);
#15175=AXIS2_PLACEMENT_3D('',#20679,#16890,#16891);
#15176=AXIS2_PLACEMENT_3D('',#20682,#16893,#16894);
#15177=AXIS2_PLACEMENT_3D('',#20683,#16895,#16896);
#15178=AXIS2_PLACEMENT_3D('',#20686,#16898,#16899);
#15179=AXIS2_PLACEMENT_3D('',#20687,#16900,#16901);
#15180=AXIS2_PLACEMENT_3D('',#20689,#16903,#16904);
#15181=AXIS2_PLACEMENT_3D('',#20692,#16906,#16907);
#15182=AXIS2_PLACEMENT_3D('',#20693,#16908,#16909);
#15183=AXIS2_PLACEMENT_3D('',#20706,#16916,#16917);
#15184=AXIS2_PLACEMENT_3D('',#20712,#16921,#16922);
#15185=AXIS2_PLACEMENT_3D('',#20716,#16925,#16926);
#15186=AXIS2_PLACEMENT_3D('',#20722,#16930,#16931);
#15187=AXIS2_PLACEMENT_3D('',#20726,#16934,#16935);
#15188=AXIS2_PLACEMENT_3D('',#20728,#16937,#16938);
#15189=AXIS2_PLACEMENT_3D('',#20730,#16940,#16941);
#15190=AXIS2_PLACEMENT_3D('',#20733,#16944,#16945);
#15191=AXIS2_PLACEMENT_3D('',#20735,#16947,#16948);
#15192=AXIS2_PLACEMENT_3D('',#20737,#16950,#16951);
#15193=AXIS2_PLACEMENT_3D('',#20740,#16953,#16954);
#15194=AXIS2_PLACEMENT_3D('',#20741,#16955,#16956);
#15195=AXIS2_PLACEMENT_3D('',#20754,#16963,#16964);
#15196=AXIS2_PLACEMENT_3D('',#20760,#16968,#16969);
#15197=AXIS2_PLACEMENT_3D('',#20763,#16971,#16972);
#15198=AXIS2_PLACEMENT_3D('',#20764,#16973,#16974);
#15199=AXIS2_PLACEMENT_3D('',#20768,#16977,#16978);
#15200=AXIS2_PLACEMENT_3D('',#20777,#16983,#16984);
#15201=AXIS2_PLACEMENT_3D('',#20783,#16988,#16989);
#15202=AXIS2_PLACEMENT_3D('',#20792,#16994,#16995);
#15203=AXIS2_PLACEMENT_3D('',#20798,#16999,#17000);
#15204=AXIS2_PLACEMENT_3D('',#20801,#17003,#17004);
#15205=AXIS2_PLACEMENT_3D('',#20804,#17007,#17008);
#15206=AXIS2_PLACEMENT_3D('',#20807,#17011,#17012);
#15207=AXIS2_PLACEMENT_3D('',#20809,#17014,#17015);
#15208=AXIS2_PLACEMENT_3D('',#20811,#17017,#17018);
#15209=AXIS2_PLACEMENT_3D('',#20813,#17020,#17021);
#15210=AXIS2_PLACEMENT_3D('',#20820,#17025,#17026);
#15211=AXIS2_PLACEMENT_3D('',#20826,#17030,#17031);
#15212=AXIS2_PLACEMENT_3D('',#20833,#17035,#17036);
#15213=AXIS2_PLACEMENT_3D('',#20839,#17040,#17041);
#15214=AXIS2_PLACEMENT_3D('',#20847,#17046,#17047);
#15215=AXIS2_PLACEMENT_3D('',#20850,#17050,#17051);
#15216=AXIS2_PLACEMENT_3D('',#20858,#17056,#17057);
#15217=AXIS2_PLACEMENT_3D('',#20860,#17059,#17060);
#15218=AXIS2_PLACEMENT_3D('',#20864,#17063,#17064);
#15219=AXIS2_PLACEMENT_3D('',#20870,#17068,#17069);
#15220=AXIS2_PLACEMENT_3D('',#20877,#17073,#17074);
#15221=AXIS2_PLACEMENT_3D('',#20883,#17078,#17079);
#15222=AXIS2_PLACEMENT_3D('',#20890,#17083,#17084);
#15223=AXIS2_PLACEMENT_3D('',#20896,#17088,#17089);
#15224=AXIS2_PLACEMENT_3D('',#20904,#17094,#17095);
#15225=AXIS2_PLACEMENT_3D('',#20907,#17098,#17099);
#15226=AXIS2_PLACEMENT_3D('',#20915,#17104,#17105);
#15227=AXIS2_PLACEMENT_3D('',#20917,#17107,#17108);
#15228=AXIS2_PLACEMENT_3D('',#20921,#17111,#17112);
#15229=AXIS2_PLACEMENT_3D('',#20927,#17116,#17117);
#15230=AXIS2_PLACEMENT_3D('',#20935,#17122,#17123);
#15231=AXIS2_PLACEMENT_3D('',#20939,#17126,#17127);
#15232=AXIS2_PLACEMENT_3D('',#20945,#17131,#17132);
#15233=AXIS2_PLACEMENT_3D('',#20954,#17137,#17138);
#15234=AXIS2_PLACEMENT_3D('',#20960,#17142,#17143);
#15235=AXIS2_PLACEMENT_3D('',#20966,#17147,#17148);
#15236=AXIS2_PLACEMENT_3D('',#20970,#17151,#17152);
#15237=AXIS2_PLACEMENT_3D('',#20976,#17156,#17157);
#15238=AXIS2_PLACEMENT_3D('',#20979,#17160,#17161);
#15239=AXIS2_PLACEMENT_3D('',#20986,#17164,#17165);
#15240=AXIS2_PLACEMENT_3D('',#21009,#17178,#17179);
#15241=AXIS2_PLACEMENT_3D('',#21011,#17181,#17182);
#15242=AXIS2_PLACEMENT_3D('',#21017,#17186,#17187);
#15243=AXIS2_PLACEMENT_3D('',#21021,#17189,#17190);
#15244=AXIS2_PLACEMENT_3D('',#21022,#17191,#17192);
#15245=AXIS2_PLACEMENT_3D('',#21023,#17193,#17194);
#15246=AXIS2_PLACEMENT_3D('',#21029,#17198,#17199);
#15247=AXIS2_PLACEMENT_3D('',#21033,#17201,#17202);
#15248=AXIS2_PLACEMENT_3D('',#21034,#17203,#17204);
#15249=AXIS2_PLACEMENT_3D('',#21035,#17205,#17206);
#15250=AXIS2_PLACEMENT_3D('',#21041,#17210,#17211);
#15251=AXIS2_PLACEMENT_3D('',#21045,#17213,#17214);
#15252=AXIS2_PLACEMENT_3D('',#21046,#17215,#17216);
#15253=AXIS2_PLACEMENT_3D('',#21047,#17217,#17218);
#15254=AXIS2_PLACEMENT_3D('',#21053,#17222,#17223);
#15255=AXIS2_PLACEMENT_3D('',#21054,#17224,#17225);
#15256=AXIS2_PLACEMENT_3D('',#21055,#17226,#17227);
#15257=AXIS2_PLACEMENT_3D('',#21056,#17228,#17229);
#15258=AXIS2_PLACEMENT_3D('',#21060,#17231,#17232);
#15259=AXIS2_PLACEMENT_3D('',#21062,#17234,#17235);
#15260=AXIS2_PLACEMENT_3D('',#21067,#17238,#17239);
#15261=AXIS2_PLACEMENT_3D('',#21068,#17240,#17241);
#15262=AXIS2_PLACEMENT_3D('',#21085,#17242,#17243);
#15263=AXIS2_PLACEMENT_3D('',#21086,#17244,#17245);
#15264=AXIS2_PLACEMENT_3D('',#21087,#17246,#17247);
#15265=AXIS2_PLACEMENT_3D('',#21091,#17250,#17251);
#15266=AXIS2_PLACEMENT_3D('',#21095,#17254,#17255);
#15267=AXIS2_PLACEMENT_3D('',#21098,#17258,#17259);
#15268=AXIS2_PLACEMENT_3D('',#21102,#17262,#17263);
#15269=AXIS2_PLACEMENT_3D('',#21104,#17264,#17265);
#15270=AXIS2_PLACEMENT_3D('',#21107,#17267,#17268);
#15271=AXIS2_PLACEMENT_3D('',#21108,#17269,#17270);
#15272=AXIS2_PLACEMENT_3D('',#21114,#17274,#17275);
#15273=AXIS2_PLACEMENT_3D('',#21116,#17276,#17277);
#15274=AXIS2_PLACEMENT_3D('',#21119,#17279,#17280);
#15275=AXIS2_PLACEMENT_3D('',#21120,#17281,#17282);
#15276=AXIS2_PLACEMENT_3D('',#21125,#17286,#17287);
#15277=AXIS2_PLACEMENT_3D('',#21128,#17289,#17290);
#15278=AXIS2_PLACEMENT_3D('',#21129,#17291,#17292);
#15279=AXIS2_PLACEMENT_3D('',#21133,#17295,#17296);
#15280=AXIS2_PLACEMENT_3D('',#21136,#17298,#17299);
#15281=AXIS2_PLACEMENT_3D('',#21137,#17300,#17301);
#15282=AXIS2_PLACEMENT_3D('',#21140,#17304,#17305);
#15283=AXIS2_PLACEMENT_3D('',#21142,#17307,#17308);
#15284=AXIS2_PLACEMENT_3D('',#21144,#17310,#17311);
#15285=AXIS2_PLACEMENT_3D('',#21146,#17313,#17314);
#15286=AXIS2_PLACEMENT_3D('',#21149,#17317,#17318);
#15287=AXIS2_PLACEMENT_3D('',#21151,#17320,#17321);
#15288=AXIS2_PLACEMENT_3D('',#21153,#17323,#17324);
#15289=AXIS2_PLACEMENT_3D('',#21155,#17326,#17327);
#15290=AXIS2_PLACEMENT_3D('',#21157,#17329,#17330);
#15291=AXIS2_PLACEMENT_3D('',#21174,#17331,#17332);
#15292=AXIS2_PLACEMENT_3D('',#21176,#17334,#17335);
#15293=AXIS2_PLACEMENT_3D('',#21177,#17336,#17337);
#15294=AXIS2_PLACEMENT_3D('',#21179,#17339,#17340);
#15295=AXIS2_PLACEMENT_3D('',#21180,#17341,#17342);
#15296=AXIS2_PLACEMENT_3D('',#21215,#17345,#17346);
#15297=AXIS2_PLACEMENT_3D('',#21219,#17348,#17349);
#15298=AXIS2_PLACEMENT_3D('',#21221,#17350,#17351);
#15299=AXIS2_PLACEMENT_3D('',#21263,#17353,#17354);
#15300=AXIS2_PLACEMENT_3D('',#21266,#17356,#17357);
#15301=AXIS2_PLACEMENT_3D('',#21304,#17360,#17361);
#15302=AXIS2_PLACEMENT_3D('',#21308,#17363,#17364);
#15303=AXIS2_PLACEMENT_3D('',#21350,#17366,#17367);
#15304=AXIS2_PLACEMENT_3D('',#21353,#17369,#17370);
#15305=AXIS2_PLACEMENT_3D('',#21354,#17371,#17372);
#15306=AXIS2_PLACEMENT_3D('',#21357,#17374,#17375);
#15307=AXIS2_PLACEMENT_3D('',#21358,#17376,#17377);
#15308=AXIS2_PLACEMENT_3D('',#21361,#17379,#17380);
#15309=AXIS2_PLACEMENT_3D('',#21362,#17381,#17382);
#15310=AXIS2_PLACEMENT_3D('',#21364,#17383,#17384);
#15311=AXIS2_PLACEMENT_3D('',#21366,#17386,#17387);
#15312=AXIS2_PLACEMENT_3D('',#21370,#17390,#17391);
#15313=AXIS2_PLACEMENT_3D('',#21371,#17392,#17393);
#15314=AXIS2_PLACEMENT_3D('',#21372,#17394,#17395);
#15315=AXIS2_PLACEMENT_3D('',#21374,#17397,#17398);
#15316=AXIS2_PLACEMENT_3D('',#21376,#17400,#17401);
#15317=AXIS2_PLACEMENT_3D('',#21377,#17402,#17403);
#15318=AXIS2_PLACEMENT_3D('',#21379,#17405,#17406);
#15319=AXIS2_PLACEMENT_3D('',#21381,#17408,#17409);
#15320=AXIS2_PLACEMENT_3D('',#21382,#17410,#17411);
#15321=AXIS2_PLACEMENT_3D('',#21384,#17413,#17414);
#15322=AXIS2_PLACEMENT_3D('',#21385,#17415,#17416);
#16749=DIRECTION('axis',(0.,0.,1.));
#16750=DIRECTION('refdir',(1.,0.,0.));
#16751=DIRECTION('center_axis',(0.707106781186549,0.707106781186546,0.));
#16752=DIRECTION('ref_axis',(0.,0.,-1.));
#16753=DIRECTION('',(0.707106781186546,-0.707106781186549,0.));
#16754=DIRECTION('',(0.,0.,1.));
#16755=DIRECTION('',(0.707106781186547,-0.707106781186548,0.));
#16756=DIRECTION('',(0.,0.,-1.));
#16757=DIRECTION('center_axis',(-1.,0.,0.));
#16758=DIRECTION('ref_axis',(0.,1.,7.40148683083438E-16));
#16759=DIRECTION('',(0.707106781186547,0.707106781186548,0.));
#16760=DIRECTION('center_axis',(-1.,0.,0.));
#16761=DIRECTION('ref_axis',(0.,1.,7.40148683083438E-16));
#16762=DIRECTION('center_axis',(1.,0.,0.));
#16763=DIRECTION('ref_axis',(0.,1.,7.40148683083438E-16));
#16764=DIRECTION('center_axis',(0.707106781186549,-0.707106781186546,0.));
#16765=DIRECTION('ref_axis',(0.,0.,-1.));
#16766=DIRECTION('',(-0.707106781186546,-0.707106781186549,0.));
#16767=DIRECTION('',(0.,0.,1.));
#16768=DIRECTION('',(0.,0.,-1.));
#16769=DIRECTION('center_axis',(0.,-1.,0.));
#16770=DIRECTION('ref_axis',(0.,0.,-1.));
#16771=DIRECTION('',(1.,0.,0.));
#16772=DIRECTION('',(0.,0.,1.));
#16773=DIRECTION('',(-1.,0.,0.));
#16774=DIRECTION('center_axis',(1.,0.,0.));
#16775=DIRECTION('ref_axis',(0.,1.,7.40148683083438E-16));
#16776=DIRECTION('',(1.,0.,0.));
#16777=DIRECTION('center_axis',(-1.,0.,0.));
#16778=DIRECTION('ref_axis',(0.,1.,7.40148683083438E-16));
#16779=DIRECTION('center_axis',(0.,1.,0.));
#16780=DIRECTION('ref_axis',(0.,0.,1.));
#16781=DIRECTION('',(1.,0.,0.));
#16782=DIRECTION('',(0.,0.,-1.));
#16783=DIRECTION('center_axis',(-0.707106781186549,0.707106781186546,0.));
#16784=DIRECTION('ref_axis',(0.,0.,1.));
#16785=DIRECTION('',(0.707106781186546,0.707106781186549,0.));
#16786=DIRECTION('',(0.,0.,1.));
#16787=DIRECTION('',(0.707106781186547,0.707106781186548,0.));
#16788=DIRECTION('center_axis',(1.,0.,0.));
#16789=DIRECTION('ref_axis',(0.,1.,7.40148683083438E-16));
#16790=DIRECTION('',(0.707106781186547,-0.707106781186548,0.));
#16791=DIRECTION('center_axis',(1.,0.,0.));
#16792=DIRECTION('ref_axis',(0.,1.,7.40148683083438E-16));
#16793=DIRECTION('center_axis',(-0.707106781186549,-0.707106781186546,0.));
#16794=DIRECTION('ref_axis',(0.,0.,1.));
#16795=DIRECTION('',(-0.707106781186546,0.707106781186549,0.));
#16796=DIRECTION('',(0.,0.,-1.));
#16797=DIRECTION('center_axis',(1.,0.,0.));
#16798=DIRECTION('ref_axis',(0.,0.,-1.));
#16799=DIRECTION('',(0.,1.,0.));
#16800=DIRECTION('',(0.,-0.866025403784439,-0.499999999999999));
#16801=DIRECTION('',(0.,-4.062597224754E-16,-1.));
#16802=DIRECTION('',(0.,0.866025403784439,-0.5));
#16803=DIRECTION('',(0.,0.866025403784439,0.5));
#16804=DIRECTION('',(0.,-1.354199074918E-16,1.));
#16805=DIRECTION('',(0.,-0.866025403784439,0.499999999999999));
#16806=DIRECTION('center_axis',(-0.707106781186549,-0.707106781186546,0.));
#16807=DIRECTION('ref_axis',(0.,0.,1.));
#16808=DIRECTION('',(-0.707106781186546,0.707106781186549,0.));
#16809=DIRECTION('',(0.,0.,1.));
#16810=DIRECTION('',(-0.707106781186546,0.707106781186549,0.));
#16811=DIRECTION('',(0.,0.,-1.));
#16812=DIRECTION('center_axis',(1.,0.,0.));
#16813=DIRECTION('ref_axis',(0.,1.,7.40148683083438E-16));
#16814=DIRECTION('',(-0.707106781186548,-0.707106781186548,0.));
#16815=DIRECTION('center_axis',(1.,0.,0.));
#16816=DIRECTION('ref_axis',(0.,1.,7.40148683083438E-16));
#16817=DIRECTION('center_axis',(-1.,0.,0.));
#16818=DIRECTION('ref_axis',(0.,1.,7.40148683083438E-16));
#16819=DIRECTION('center_axis',(-0.707106781186549,0.707106781186546,0.));
#16820=DIRECTION('ref_axis',(0.,0.,1.));
#16821=DIRECTION('',(0.707106781186546,0.707106781186549,0.));
#16822=DIRECTION('',(0.,0.,1.));
#16823=DIRECTION('',(0.,0.,-1.));
#16824=DIRECTION('center_axis',(0.,1.,0.));
#16825=DIRECTION('ref_axis',(0.,0.,-1.));
#16826=DIRECTION('',(-1.,0.,0.));
#16827=DIRECTION('',(0.,0.,1.));
#16828=DIRECTION('',(1.,0.,0.));
#16829=DIRECTION('center_axis',(-1.,0.,0.));
#16830=DIRECTION('ref_axis',(0.,1.,7.40148683083438E-16));
#16831=DIRECTION('',(-1.,0.,0.));
#16832=DIRECTION('center_axis',(1.,0.,0.));
#16833=DIRECTION('ref_axis',(0.,1.,7.40148683083438E-16));
#16834=DIRECTION('center_axis',(0.,-1.,0.));
#16835=DIRECTION('ref_axis',(0.,0.,1.));
#16836=DIRECTION('',(-1.,0.,0.));
#16837=DIRECTION('',(0.,0.,-1.));
#16838=DIRECTION('center_axis',(0.577350269189626,-0.577350269189625,0.577350269189626));
#16839=DIRECTION('ref_axis',(0.707106781186548,0.,-0.707106781186548));
#16840=DIRECTION('',(0.,0.707106781186549,0.707106781186546));
#16841=DIRECTION('',(-0.707106781186546,-0.707106781186549,0.));
#16842=DIRECTION('',(0.707106781186548,0.,-0.707106781186548));
#16843=DIRECTION('center_axis',(0.707106781186549,-0.707106781186546,0.));
#16844=DIRECTION('ref_axis',(0.,0.,-1.));
#16845=DIRECTION('',(-0.707106781186546,-0.707106781186549,0.));
#16846=DIRECTION('',(0.,0.,1.));
#16847=DIRECTION('',(0.,0.,-1.));
#16848=DIRECTION('center_axis',(0.707106781186548,0.,0.707106781186548));
#16849=DIRECTION('ref_axis',(0.707106781186548,0.,-0.707106781186548));
#16850=DIRECTION('',(-0.577350269189627,-0.577350269189624,0.577350269189627));
#16851=DIRECTION('',(0.,-1.,0.));
#16852=DIRECTION('',(0.,1.,0.));
#16853=DIRECTION('',(-0.577350269189625,0.577350269189628,0.577350269189625));
#16854=DIRECTION('center_axis',(0.,-0.707106781186546,0.707106781186549));
#16855=DIRECTION('ref_axis',(1.,0.,0.));
#16856=DIRECTION('',(0.577350269189626,-0.577350269189627,-0.577350269189625));
#16857=DIRECTION('',(1.,0.,0.));
#16858=DIRECTION('',(-1.,0.,0.));
#16859=DIRECTION('',(-0.577350269189627,-0.577350269189626,-0.577350269189624));
#16860=DIRECTION('center_axis',(1.,0.,0.));
#16861=DIRECTION('ref_axis',(0.,1.,0.));
#16862=DIRECTION('',(0.,-1.,0.));
#16863=DIRECTION('',(0.,0.,-1.));
#16864=DIRECTION('center_axis',(0.,-1.,0.));
#16865=DIRECTION('ref_axis',(1.,0.,0.));
#16866=DIRECTION('',(0.,0.,1.));
#16867=DIRECTION('',(-1.,0.,0.));
#16868=DIRECTION('center_axis',(-0.707106781186548,-0.707106781186547,0.));
#16869=DIRECTION('ref_axis',(0.,0.,1.));
#16870=DIRECTION('',(-0.577350269189625,0.577350269189627,-0.577350269189625));
#16871=DIRECTION('',(0.,0.,-1.));
#16872=DIRECTION('',(-0.707106781186547,0.707106781186548,0.));
#16873=DIRECTION('center_axis',(1.,0.,0.));
#16874=DIRECTION('ref_axis',(0.,0.,-1.));
#16875=DIRECTION('center_axis',(1.,0.,0.));
#16876=DIRECTION('ref_axis',(0.,0.,-1.));
#16877=DIRECTION('',(-0.707106781186548,8.65956056235493E-17,-0.707106781186548));
#16878=DIRECTION('center_axis',(-1.,0.,0.));
#16879=DIRECTION('ref_axis',(0.,0.,-1.));
#16880=DIRECTION('center_axis',(-1.,0.,0.));
#16881=DIRECTION('ref_axis',(0.,0.,-1.));
#16882=DIRECTION('',(-1.,0.,0.));
#16883=DIRECTION('center_axis',(1.,0.,0.));
#16884=DIRECTION('ref_axis',(0.,0.,-1.));
#16885=DIRECTION('center_axis',(1.,0.,0.));
#16886=DIRECTION('ref_axis',(0.,0.,-1.));
#16887=DIRECTION('',(0.,-1.,0.));
#16888=DIRECTION('center_axis',(-1.,0.,0.));
#16889=DIRECTION('ref_axis',(0.,0.,-1.));
#16890=DIRECTION('center_axis',(-1.,0.,0.));
#16891=DIRECTION('ref_axis',(0.,0.,-1.));
#16892=DIRECTION('',(0.707106781186548,-8.65956056235493E-17,-0.707106781186548));
#16893=DIRECTION('center_axis',(1.,0.,0.));
#16894=DIRECTION('ref_axis',(0.,0.,-1.));
#16895=DIRECTION('center_axis',(1.,0.,0.));
#16896=DIRECTION('ref_axis',(0.,0.,-1.));
#16897=DIRECTION('',(1.,0.,0.));
#16898=DIRECTION('center_axis',(-1.,0.,0.));
#16899=DIRECTION('ref_axis',(0.,0.,-1.));
#16900=DIRECTION('center_axis',(1.,0.,0.));
#16901=DIRECTION('ref_axis',(0.,0.,-1.));
#16902=DIRECTION('',(0.,1.,0.));
#16903=DIRECTION('center_axis',(-1.,0.,0.));
#16904=DIRECTION('ref_axis',(0.,0.,-1.));
#16905=DIRECTION('',(-0.707106781186548,-8.65956056235493E-17,0.707106781186548));
#16906=DIRECTION('center_axis',(-1.,0.,0.));
#16907=DIRECTION('ref_axis',(0.,0.,-1.));
#16908=DIRECTION('center_axis',(1.,0.,0.));
#16909=DIRECTION('ref_axis',(0.,0.,-1.));
#16910=DIRECTION('',(0.,4.062597224754E-16,1.));
#16911=DIRECTION('',(0.,0.866025403784439,0.499999999999999));
#16912=DIRECTION('',(0.,0.866025403784439,-0.499999999999999));
#16913=DIRECTION('',(0.,1.354199074918E-16,-1.));
#16914=DIRECTION('',(0.,-0.866025403784439,-0.5));
#16915=DIRECTION('',(0.,-0.866025403784439,0.5));
#16916=DIRECTION('center_axis',(-0.70710678118655,0.353553390593272,-0.612372435695792));
#16917=DIRECTION('ref_axis',(-0.654653670707974,0.,0.755928946018457));
#16918=DIRECTION('',(0.654653670707975,-3.98171761111234E-16,-0.755928946018456));
#16919=DIRECTION('',(0.,-0.866025403784439,-0.5));
#16920=DIRECTION('',(0.654653670707976,0.654653670707976,-0.377964473009231));
#16921=DIRECTION('center_axis',(-0.70710678118655,-0.353553390593272,-0.612372435695792));
#16922=DIRECTION('ref_axis',(-0.654653670707974,0.,0.755928946018457));
#16923=DIRECTION('',(0.654653670707975,-0.654653670707977,-0.377964473009231));
#16924=DIRECTION('',(0.,-0.866025403784439,0.5));
#16925=DIRECTION('center_axis',(-0.707106781186554,-0.35355339059327,0.612372435695789));
#16926=DIRECTION('ref_axis',(0.654653670707971,0.,0.75592894601846));
#16927=DIRECTION('',(0.654653670707972,-4.61997734366925E-15,0.755928946018459));
#16928=DIRECTION('',(0.,0.866025403784439,0.499999999999999));
#16929=DIRECTION('',(-0.654653670707974,0.654653670707975,-0.377964473009236));
#16930=DIRECTION('center_axis',(-0.707106781186551,0.353553390593272,0.612372435695792));
#16931=DIRECTION('ref_axis',(0.654653670707974,0.,0.755928946018457));
#16932=DIRECTION('',(0.,0.866025403784439,-0.499999999999999));
#16933=DIRECTION('',(0.654653670707974,0.654653670707975,0.377964473009236));
#16934=DIRECTION('center_axis',(-0.707106781186548,-0.707106781186547,2.8726900468532E-16));
#16935=DIRECTION('ref_axis',(4.062597224754E-16,0.,1.));
#16936=DIRECTION('',(0.,4.062597224754E-16,1.));
#16937=DIRECTION('center_axis',(-0.707106781186548,0.707106781186547,9.57563348951068E-17));
#16938=DIRECTION('ref_axis',(1.354199074918E-16,0.,1.));
#16939=DIRECTION('',(0.,1.354199074918E-16,-1.));
#16940=DIRECTION('center_axis',(0.,0.5,0.866025403784439));
#16941=DIRECTION('ref_axis',(0.,-0.866025403784439,0.5));
#16942=DIRECTION('',(1.,0.,0.));
#16943=DIRECTION('',(1.,0.,0.));
#16944=DIRECTION('center_axis',(0.,1.,-4.062597224754E-16));
#16945=DIRECTION('ref_axis',(0.,4.062597224754E-16,1.));
#16946=DIRECTION('',(1.,0.,0.));
#16947=DIRECTION('center_axis',(0.,0.499999999999999,-0.866025403784439));
#16948=DIRECTION('ref_axis',(0.,0.866025403784439,0.499999999999999));
#16949=DIRECTION('',(1.,0.,0.));
#16950=DIRECTION('center_axis',(1.,0.,0.));
#16951=DIRECTION('ref_axis',(0.,0.,-1.));
#16952=DIRECTION('',(0.707106781186548,8.65956056235493E-17,0.707106781186548));
#16953=DIRECTION('center_axis',(1.,0.,0.));
#16954=DIRECTION('ref_axis',(0.,0.,-1.));
#16955=DIRECTION('center_axis',(-1.,0.,0.));
#16956=DIRECTION('ref_axis',(0.,0.,1.));
#16957=DIRECTION('',(0.,-4.062597224754E-16,-1.));
#16958=DIRECTION('',(0.,0.866025403784439,-0.5));
#16959=DIRECTION('',(0.,0.866025403784439,0.5));
#16960=DIRECTION('',(0.,-1.354199074918E-16,1.));
#16961=DIRECTION('',(0.,-0.866025403784439,0.499999999999999));
#16962=DIRECTION('',(0.,-0.866025403784439,-0.499999999999999));
#16963=DIRECTION('center_axis',(0.707106781186549,0.707106781186546,0.));
#16964=DIRECTION('ref_axis',(0.,0.,-1.));
#16965=DIRECTION('',(0.707106781186546,-0.707106781186549,0.));
#16966=DIRECTION('',(0.707106781186547,-0.707106781186548,0.));
#16967=DIRECTION('',(0.,0.,-1.));
#16968=DIRECTION('center_axis',(-1.,0.,0.));
#16969=DIRECTION('ref_axis',(0.,1.,7.40148683083438E-16));
#16970=DIRECTION('',(0.707106781186547,0.707106781186548,0.));
#16971=DIRECTION('center_axis',(-1.,0.,0.));
#16972=DIRECTION('ref_axis',(0.,1.,7.40148683083438E-16));
#16973=DIRECTION('center_axis',(0.707106781186549,-0.707106781186546,0.));
#16974=DIRECTION('ref_axis',(0.,0.,-1.));
#16975=DIRECTION('',(-0.707106781186546,-0.707106781186549,0.));
#16976=DIRECTION('',(0.,0.,1.));
#16977=DIRECTION('center_axis',(0.70710678118655,0.353553390593272,0.612372435695793));
#16978=DIRECTION('ref_axis',(0.654653670707975,0.,-0.755928946018457));
#16979=DIRECTION('',(0.,0.866025403784439,-0.499999999999999));
#16980=DIRECTION('',(-0.654653670707975,-3.8931657652939E-15,0.755928946018456));
#16981=DIRECTION('',(0.,-0.866025403784439,0.499999999999999));
#16982=DIRECTION('',(-0.654653670707975,0.654653670707977,0.377964473009231));
#16983=DIRECTION('center_axis',(0.707106781186551,-0.353553390593272,0.612372435695792));
#16984=DIRECTION('ref_axis',(0.654653670707974,0.,-0.755928946018457));
#16985=DIRECTION('',(0.,0.866025403784439,0.499999999999999));
#16986=DIRECTION('',(-0.654653670707974,-0.654653670707975,0.377964473009236));
#16987=DIRECTION('',(0.,-0.866025403784439,-0.499999999999999));
#16988=DIRECTION('center_axis',(0.70710678118655,-0.353553390593272,-0.612372435695792));
#16989=DIRECTION('ref_axis',(-0.654653670707974,0.,-0.755928946018457));
#16990=DIRECTION('',(0.,-0.866025403784439,0.5));
#16991=DIRECTION('',(-0.654653670707975,3.28639817264138E-16,-0.755928946018456));
#16992=DIRECTION('',(0.,0.866025403784439,-0.5));
#16993=DIRECTION('',(0.654653670707975,0.654653670707977,0.377964473009231));
#16994=DIRECTION('center_axis',(0.70710678118655,0.353553390593272,-0.612372435695792));
#16995=DIRECTION('ref_axis',(-0.654653670707974,0.,-0.755928946018457));
#16996=DIRECTION('',(0.,0.866025403784439,0.5));
#16997=DIRECTION('',(0.,-0.866025403784439,-0.5));
#16998=DIRECTION('',(-0.654653670707975,0.654653670707977,-0.377964473009231));
#16999=DIRECTION('center_axis',(0.707106781186548,-0.707106781186547,2.8726900468532E-16));
#17000=DIRECTION('ref_axis',(4.062597224754E-16,0.,-1.));
#17001=DIRECTION('',(0.,4.062597224754E-16,1.));
#17002=DIRECTION('',(0.,-4.062597224754E-16,-1.));
#17003=DIRECTION('center_axis',(0.707106781186548,0.707106781186547,9.57563348951068E-17));
#17004=DIRECTION('ref_axis',(1.354199074918E-16,0.,-1.));
#17005=DIRECTION('',(0.,-1.354199074918E-16,1.));
#17006=DIRECTION('',(0.,1.354199074918E-16,-1.));
#17007=DIRECTION('center_axis',(0.,0.499999999999999,-0.866025403784439));
#17008=DIRECTION('ref_axis',(0.,-0.866025403784439,-0.499999999999999));
#17009=DIRECTION('',(-1.,0.,0.));
#17010=DIRECTION('',(-1.,0.,0.));
#17011=DIRECTION('center_axis',(0.,1.,-4.062597224754E-16));
#17012=DIRECTION('ref_axis',(0.,-4.062597224754E-16,-1.));
#17013=DIRECTION('',(-1.,0.,0.));
#17014=DIRECTION('center_axis',(0.,0.5,0.866025403784439));
#17015=DIRECTION('ref_axis',(0.,0.866025403784439,-0.5));
#17016=DIRECTION('',(-1.,0.,0.));
#17017=DIRECTION('center_axis',(1.,0.,0.));
#17018=DIRECTION('ref_axis',(0.,0.,-1.));
#17019=DIRECTION('',(0.,-1.,0.));
#17020=DIRECTION('center_axis',(-0.577350269189626,-0.577350269189625,0.577350269189627));
#17021=DIRECTION('ref_axis',(0.707106781186548,0.,0.707106781186547));
#17022=DIRECTION('',(0.707106781186548,7.8504622934189E-16,0.707106781186548));
#17023=DIRECTION('',(-0.707106781186547,0.707106781186548,0.));
#17024=DIRECTION('',(0.,-0.707106781186549,-0.707106781186546));
#17025=DIRECTION('center_axis',(-0.707106781186548,-0.707106781186547,0.));
#17026=DIRECTION('ref_axis',(0.,0.,1.));
#17027=DIRECTION('',(-0.707106781186547,0.707106781186548,0.));
#17028=DIRECTION('',(0.,0.,1.));
#17029=DIRECTION('',(0.,0.,-1.));
#17030=DIRECTION('center_axis',(0.577350269189625,-0.577350269189625,0.577350269189627));
#17031=DIRECTION('ref_axis',(0.707106781186549,0.,-0.707106781186546));
#17032=DIRECTION('',(0.,0.707106781186549,0.707106781186546));
#17033=DIRECTION('',(-0.707106781186548,-0.707106781186547,0.));
#17034=DIRECTION('',(0.707106781186549,0.,-0.707106781186546));
#17035=DIRECTION('center_axis',(0.707106781186547,-0.707106781186548,0.));
#17036=DIRECTION('ref_axis',(0.,0.,-1.));
#17037=DIRECTION('',(-0.707106781186548,-0.707106781186547,0.));
#17038=DIRECTION('',(0.,0.,1.));
#17039=DIRECTION('',(0.,0.,-1.));
#17040=DIRECTION('center_axis',(0.707106781186546,0.,0.707106781186549));
#17041=DIRECTION('ref_axis',(0.707106781186549,0.,-0.707106781186546));
#17042=DIRECTION('',(-0.577350269189628,-0.577350269189623,0.577350269189626));
#17043=DIRECTION('',(0.,-1.,0.));
#17044=DIRECTION('',(0.,1.,0.));
#17045=DIRECTION('',(-0.577350269189627,0.577350269189625,0.577350269189625));
#17046=DIRECTION('center_axis',(0.,-0.707106781186546,0.707106781186549));
#17047=DIRECTION('ref_axis',(1.,0.,0.));
#17048=DIRECTION('',(-1.,0.,0.));
#17049=DIRECTION('',(1.,0.,0.));
#17050=DIRECTION('center_axis',(-0.707106781186548,0.,0.707106781186548));
#17051=DIRECTION('ref_axis',(0.707106781186548,0.,0.707106781186548));
#17052=DIRECTION('',(-0.577350269189627,-0.577350269189624,-0.577350269189627));
#17053=DIRECTION('',(0.,-1.,0.));
#17054=DIRECTION('',(0.,1.,0.));
#17055=DIRECTION('',(-0.577350269189627,0.577350269189624,-0.577350269189627));
#17056=DIRECTION('center_axis',(0.,-1.,0.));
#17057=DIRECTION('ref_axis',(1.,0.,0.));
#17058=DIRECTION('',(-1.,0.,0.));
#17059=DIRECTION('center_axis',(-1.,0.,0.));
#17060=DIRECTION('ref_axis',(0.,-1.,0.));
#17061=DIRECTION('',(0.,0.,1.));
#17062=DIRECTION('',(0.,1.,0.));
#17063=DIRECTION('center_axis',(-0.707106781186546,0.707106781186549,0.));
#17064=DIRECTION('ref_axis',(0.,0.,1.));
#17065=DIRECTION('',(0.577350269189627,0.577350269189624,-0.577350269189627));
#17066=DIRECTION('',(0.,0.,-1.));
#17067=DIRECTION('',(0.577350269189625,0.577350269189622,-0.57735026918963));
#17068=DIRECTION('center_axis',(-0.577350269189625,-0.577350269189626,0.577350269189627));
#17069=DIRECTION('ref_axis',(0.707106781186549,0.,0.707106781186546));
#17070=DIRECTION('',(0.707106781186549,7.85046229341889E-16,0.707106781186546));
#17071=DIRECTION('',(-0.707106781186548,0.707106781186547,0.));
#17072=DIRECTION('',(7.85046229341889E-16,-0.707106781186549,-0.707106781186546));
#17073=DIRECTION('center_axis',(-0.707106781186547,-0.707106781186548,0.));
#17074=DIRECTION('ref_axis',(0.,0.,1.));
#17075=DIRECTION('',(-0.707106781186548,0.707106781186547,0.));
#17076=DIRECTION('',(0.,0.,1.));
#17077=DIRECTION('',(0.,0.,-1.));
#17078=DIRECTION('center_axis',(0.577350269189625,-0.577350269189626,0.577350269189627));
#17079=DIRECTION('ref_axis',(0.707106781186549,0.,-0.707106781186546));
#17080=DIRECTION('',(0.,0.707106781186549,0.707106781186546));
#17081=DIRECTION('',(-0.707106781186548,-0.707106781186547,0.));
#17082=DIRECTION('',(0.707106781186549,0.,-0.707106781186546));
#17083=DIRECTION('center_axis',(0.707106781186547,-0.707106781186548,0.));
#17084=DIRECTION('ref_axis',(0.,0.,-1.));
#17085=DIRECTION('',(-0.707106781186548,-0.707106781186547,0.));
#17086=DIRECTION('',(0.,0.,1.));
#17087=DIRECTION('',(0.,0.,-1.));
#17088=DIRECTION('center_axis',(0.707106781186546,0.,0.707106781186549));
#17089=DIRECTION('ref_axis',(0.707106781186549,0.,-0.707106781186546));
#17090=DIRECTION('',(-0.577350269189628,-0.577350269189623,0.577350269189626));
#17091=DIRECTION('',(0.,-1.,0.));
#17092=DIRECTION('',(0.,1.,0.));
#17093=DIRECTION('',(-0.577350269189628,0.577350269189624,0.577350269189626));
#17094=DIRECTION('center_axis',(0.,-0.707106781186546,0.707106781186549));
#17095=DIRECTION('ref_axis',(1.,0.,0.));
#17096=DIRECTION('',(-1.,0.,0.));
#17097=DIRECTION('',(1.,0.,0.));
#17098=DIRECTION('center_axis',(-0.707106781186546,0.,0.707106781186549));
#17099=DIRECTION('ref_axis',(0.707106781186549,0.,0.707106781186546));
#17100=DIRECTION('',(-0.577350269189626,-0.577350269189627,-0.577350269189624));
#17101=DIRECTION('',(0.,-1.,0.));
#17102=DIRECTION('',(0.,1.,0.));
#17103=DIRECTION('',(-0.577350269189628,0.577350269189623,-0.577350269189626));
#17104=DIRECTION('center_axis',(0.,-1.,0.));
#17105=DIRECTION('ref_axis',(1.,0.,0.));
#17106=DIRECTION('',(-1.,0.,0.));
#17107=DIRECTION('center_axis',(-1.,0.,0.));
#17108=DIRECTION('ref_axis',(0.,-1.,0.));
#17109=DIRECTION('',(0.,0.,1.));
#17110=DIRECTION('',(0.,1.,0.));
#17111=DIRECTION('center_axis',(-0.707106781186548,0.707106781186547,0.));
#17112=DIRECTION('ref_axis',(0.,0.,1.));
#17113=DIRECTION('',(0.577350269189624,0.577350269189625,-0.577350269189628));
#17114=DIRECTION('',(0.,0.,-1.));
#17115=DIRECTION('',(0.577350269189622,0.577350269189624,-0.577350269189631));
#17116=DIRECTION('center_axis',(-0.707106781186546,0.,0.707106781186549));
#17117=DIRECTION('ref_axis',(0.707106781186549,0.,0.707106781186546));
#17118=DIRECTION('',(0.,1.,0.));
#17119=DIRECTION('',(-0.577350269189628,0.577350269189623,-0.577350269189626));
#17120=DIRECTION('',(-0.577350269189627,-0.577350269189627,-0.577350269189624));
#17121=DIRECTION('',(0.,-1.,0.));
#17122=DIRECTION('center_axis',(-1.,0.,0.));
#17123=DIRECTION('ref_axis',(0.,-1.,0.));
#17124=DIRECTION('',(0.,0.,1.));
#17125=DIRECTION('',(0.,1.,0.));
#17126=DIRECTION('center_axis',(-0.707106781186548,0.707106781186548,0.));
#17127=DIRECTION('ref_axis',(0.,0.,1.));
#17128=DIRECTION('',(0.577350269189625,0.577350269189625,-0.577350269189627));
#17129=DIRECTION('',(0.,0.,-1.));
#17130=DIRECTION('',(0.577350269189623,0.577350269189623,-0.577350269189631));
#17131=DIRECTION('center_axis',(0.,0.707106781186552,0.707106781186543));
#17132=DIRECTION('ref_axis',(1.,0.,0.));
#17133=DIRECTION('',(1.,0.,0.));
#17134=DIRECTION('',(-0.577350269189618,-0.577350269189626,0.577350269189633));
#17135=DIRECTION('',(-1.,0.,0.));
#17136=DIRECTION('',(0.577350269189625,-0.577350269189622,0.57735026918963));
#17137=DIRECTION('center_axis',(0.707106781186546,0.707106781186549,0.));
#17138=DIRECTION('ref_axis',(0.,0.,-1.));
#17139=DIRECTION('',(0.,0.,1.));
#17140=DIRECTION('',(-0.577350269189625,0.577350269189622,0.57735026918963));
#17141=DIRECTION('',(0.,0.,-1.));
#17142=DIRECTION('center_axis',(0.,0.,-1.));
#17143=DIRECTION('ref_axis',(1.,0.,0.));
#17144=DIRECTION('',(0.,-1.,0.));
#17145=DIRECTION('',(1.,0.,0.));
#17146=DIRECTION('',(0.,-1.,0.));
#17147=DIRECTION('center_axis',(-1.,0.,0.));
#17148=DIRECTION('ref_axis',(0.,0.,-1.));
#17149=DIRECTION('',(0.,-1.,0.));
#17150=DIRECTION('',(0.,0.,-1.));
#17151=DIRECTION('center_axis',(-0.707106781186552,0.707106781186543,0.));
#17152=DIRECTION('ref_axis',(0.,0.,1.));
#17153=DIRECTION('',(0.,0.,-1.));
#17154=DIRECTION('',(0.,0.,1.));
#17155=DIRECTION('',(0.577350269189618,0.577350269189626,0.577350269189633));
#17156=DIRECTION('center_axis',(0.,0.707106781186552,-0.707106781186543));
#17157=DIRECTION('ref_axis',(-1.,0.,0.));
#17158=DIRECTION('',(-1.,0.,0.));
#17159=DIRECTION('',(1.,0.,0.));
#17160=DIRECTION('center_axis',(0.,1.,0.));
#17161=DIRECTION('ref_axis',(-1.,0.,0.));
#17162=DIRECTION('',(1.,0.,0.));
#17163=DIRECTION('',(0.,0.,-1.));
#17164=DIRECTION('center_axis',(0.,1.,0.));
#17165=DIRECTION('ref_axis',(1.,0.,0.));
#17166=DIRECTION('',(0.,0.,-1.));
#17167=DIRECTION('',(-1.,0.,0.));
#17168=DIRECTION('',(-1.,0.,0.));
#17169=DIRECTION('',(0.,0.,1.));
#17170=DIRECTION('',(-1.,0.,0.));
#17171=DIRECTION('',(-1.,0.,0.));
#17172=DIRECTION('',(0.,0.,1.));
#17173=DIRECTION('',(-1.,0.,0.));
#17174=DIRECTION('',(-1.,0.,0.));
#17175=DIRECTION('',(0.,0.,1.));
#17176=DIRECTION('',(-1.,0.,0.));
#17177=DIRECTION('',(0.,0.,1.));
#17178=DIRECTION('center_axis',(0.,1.,0.));
#17179=DIRECTION('ref_axis',(-1.,0.,0.));
#17180=DIRECTION('',(0.,0.,1.));
#17181=DIRECTION('center_axis',(0.,0.707106781186546,-0.707106781186549));
#17182=DIRECTION('ref_axis',(-1.,0.,0.));
#17183=DIRECTION('',(-6.28036983473511E-15,0.707106781186549,0.707106781186546));
#17184=DIRECTION('',(0.,-0.707106781186549,-0.707106781186546));
#17185=DIRECTION('',(-1.,0.,0.));
#17186=DIRECTION('center_axis',(0.,0.,1.));
#17187=DIRECTION('ref_axis',(-0.707106781186546,0.707106781186548,0.));
#17188=DIRECTION('',(-0.707106781186544,-1.57009245868379E-15,0.707106781186551));
#17189=DIRECTION('center_axis',(0.,0.,-1.));
#17190=DIRECTION('ref_axis',(-0.707106781186546,0.707106781186549,0.));
#17191=DIRECTION('center_axis',(0.,0.,1.));
#17192=DIRECTION('ref_axis',(-0.707106781186546,0.707106781186549,0.));
#17193=DIRECTION('center_axis',(-0.707106781186548,0.,-0.707106781186548));
#17194=DIRECTION('ref_axis',(-0.707106781186548,0.,0.707106781186548));
#17195=DIRECTION('',(-0.707106781186548,0.,0.707106781186548));
#17196=DIRECTION('',(0.,1.,0.));
#17197=DIRECTION('',(0.,-1.,0.));
#17198=DIRECTION('center_axis',(0.,0.,1.));
#17199=DIRECTION('ref_axis',(-0.707106781186549,-0.707106781186546,0.));
#17200=DIRECTION('',(0.,-0.707106781186549,0.707106781186546));
#17201=DIRECTION('center_axis',(0.,0.,-1.));
#17202=DIRECTION('ref_axis',(-0.707106781186549,-0.707106781186546,0.));
#17203=DIRECTION('center_axis',(0.,0.,1.));
#17204=DIRECTION('ref_axis',(-0.707106781186549,-0.707106781186546,0.));
#17205=DIRECTION('center_axis',(0.,-0.707106781186546,-0.707106781186549));
#17206=DIRECTION('ref_axis',(-1.,0.,0.));
#17207=DIRECTION('',(0.,-0.707106781186549,0.707106781186546));
#17208=DIRECTION('',(-1.,0.,0.));
#17209=DIRECTION('',(1.,0.,0.));
#17210=DIRECTION('center_axis',(0.,0.,1.));
#17211=DIRECTION('ref_axis',(0.707106781186549,-0.707106781186546,0.));
#17212=DIRECTION('',(0.707106781186554,0.,0.707106781186541));
#17213=DIRECTION('center_axis',(0.,0.,-1.));
#17214=DIRECTION('ref_axis',(0.707106781186549,-0.707106781186546,0.));
#17215=DIRECTION('center_axis',(0.,0.,1.));
#17216=DIRECTION('ref_axis',(0.707106781186549,-0.707106781186546,0.));
#17217=DIRECTION('center_axis',(0.707106781186548,0.,-0.707106781186548));
#17218=DIRECTION('ref_axis',(-0.707106781186548,0.,-0.707106781186548));
#17219=DIRECTION('',(0.707106781186548,0.,0.707106781186548));
#17220=DIRECTION('',(0.,-1.,0.));
#17221=DIRECTION('',(0.,1.,0.));
#17222=DIRECTION('center_axis',(0.,0.,1.));
#17223=DIRECTION('ref_axis',(0.707106781186548,0.707106781186547,0.));
#17224=DIRECTION('center_axis',(0.,0.,-1.));
#17225=DIRECTION('ref_axis',(0.707106781186548,0.707106781186547,0.));
#17226=DIRECTION('center_axis',(0.,0.,1.));
#17227=DIRECTION('ref_axis',(0.707106781186548,0.707106781186547,0.));
#17228=DIRECTION('center_axis',(0.,0.,1.));
#17229=DIRECTION('ref_axis',(0.707106781186549,-0.707106781186546,0.));
#17230=DIRECTION('',(0.,0.,1.));
#17231=DIRECTION('center_axis',(0.,0.,1.));
#17232=DIRECTION('ref_axis',(0.707106781186549,-0.707106781186546,0.));
#17233=DIRECTION('',(0.,0.,-1.));
#17234=DIRECTION('center_axis',(1.,0.,0.));
#17235=DIRECTION('ref_axis',(0.,1.,0.));
#17236=DIRECTION('',(0.,0.,-1.));
#17237=DIRECTION('',(0.,1.,0.));
#17238=DIRECTION('center_axis',(1.,0.,0.));
#17239=DIRECTION('ref_axis',(0.,0.,-1.));
#17240=DIRECTION('center_axis',(0.,0.,1.));
#17241=DIRECTION('ref_axis',(0.707106781186548,0.707106781186547,0.));
#17242=DIRECTION('center_axis',(0.,0.,1.));
#17243=DIRECTION('ref_axis',(0.707106781186548,0.707106781186547,0.));
#17244=DIRECTION('center_axis',(0.,0.,1.));
#17245=DIRECTION('ref_axis',(1.,0.,0.));
#17246=DIRECTION('center_axis',(0.,0.707106781186552,0.707106781186543));
#17247=DIRECTION('ref_axis',(1.,0.,0.));
#17248=DIRECTION('',(1.,0.,0.));
#17249=DIRECTION('',(0.577350269189626,-0.577350269189622,0.57735026918963));
#17250=DIRECTION('center_axis',(0.,0.707106781186552,0.707106781186543));
#17251=DIRECTION('ref_axis',(1.,0.,0.));
#17252=DIRECTION('',(0.577350269189625,-0.577350269189622,0.57735026918963));
#17253=DIRECTION('',(1.,0.,0.));
#17254=DIRECTION('center_axis',(0.707106781186546,0.707106781186549,0.));
#17255=DIRECTION('ref_axis',(0.,0.,-1.));
#17256=DIRECTION('',(0.,0.,-1.));
#17257=DIRECTION('',(0.577350269189627,-0.577350269189624,0.577350269189627));
#17258=DIRECTION('center_axis',(0.,0.707106781186552,0.707106781186543));
#17259=DIRECTION('ref_axis',(1.,0.,0.));
#17260=DIRECTION('',(6.28036983473505E-15,-0.707106781186543,0.707106781186552));
#17261=DIRECTION('',(1.,0.,0.));
#17262=DIRECTION('center_axis',(0.,0.,-1.));
#17263=DIRECTION('ref_axis',(-0.707106781186546,0.707106781186548,0.));
#17264=DIRECTION('center_axis',(0.,0.,1.));
#17265=DIRECTION('ref_axis',(-0.707106781186546,0.707106781186549,0.));
#17266=DIRECTION('',(0.707106781186544,1.57009245868379E-15,0.707106781186551));
#17267=DIRECTION('center_axis',(0.,0.,-1.));
#17268=DIRECTION('ref_axis',(-0.707106781186546,0.707106781186549,0.));
#17269=DIRECTION('center_axis',(-0.707106781186554,0.,0.707106781186541));
#17270=DIRECTION('ref_axis',(0.707106781186541,0.,0.707106781186554));
#17271=DIRECTION('',(0.707106781186541,0.,0.707106781186554));
#17272=DIRECTION('',(0.,1.,0.));
#17273=DIRECTION('',(0.,-1.,0.));
#17274=DIRECTION('center_axis',(0.,0.,-1.));
#17275=DIRECTION('ref_axis',(-0.707106781186549,-0.707106781186546,0.));
#17276=DIRECTION('center_axis',(0.,0.,1.));
#17277=DIRECTION('ref_axis',(-0.707106781186549,-0.707106781186546,0.));
#17278=DIRECTION('',(0.,0.707106781186549,0.707106781186546));
#17279=DIRECTION('center_axis',(0.,0.,-1.));
#17280=DIRECTION('ref_axis',(-0.707106781186549,-0.707106781186546,0.));
#17281=DIRECTION('center_axis',(0.,-0.707106781186552,0.707106781186543));
#17282=DIRECTION('ref_axis',(1.,0.,0.));
#17283=DIRECTION('',(0.,0.707106781186543,0.707106781186552));
#17284=DIRECTION('',(-1.,0.,0.));
#17285=DIRECTION('',(1.,0.,0.));
#17286=DIRECTION('center_axis',(0.,0.,-1.));
#17287=DIRECTION('ref_axis',(0.707106781186549,-0.707106781186546,0.));
#17288=DIRECTION('',(-0.707106781186554,0.,0.707106781186541));
#17289=DIRECTION('center_axis',(0.,0.,-1.));
#17290=DIRECTION('ref_axis',(0.707106781186549,-0.707106781186546,0.));
#17291=DIRECTION('center_axis',(0.707106781186554,0.,0.707106781186541));
#17292=DIRECTION('ref_axis',(0.707106781186541,0.,-0.707106781186554));
#17293=DIRECTION('',(-0.707106781186541,0.,0.707106781186554));
#17294=DIRECTION('',(0.,-1.,0.));
#17295=DIRECTION('center_axis',(0.,0.,-1.));
#17296=DIRECTION('ref_axis',(0.707106781186548,0.707106781186547,0.));
#17297=DIRECTION('',(0.,-0.70710678118655,0.707106781186545));
#17298=DIRECTION('center_axis',(0.,0.,-1.));
#17299=DIRECTION('ref_axis',(0.707106781186548,0.707106781186547,0.));
#17300=DIRECTION('center_axis',(0.,0.707106781186552,0.707106781186543));
#17301=DIRECTION('ref_axis',(1.,0.,0.));
#17302=DIRECTION('',(1.,0.,0.));
#17303=DIRECTION('',(0.577350269189622,-0.577350269189624,0.577350269189632));
#17304=DIRECTION('center_axis',(0.707106781186549,0.707106781186546,0.));
#17305=DIRECTION('ref_axis',(0.,0.,-1.));
#17306=DIRECTION('',(0.577350269189623,-0.577350269189626,0.577350269189628));
#17307=DIRECTION('center_axis',(0.,0.707106781186549,0.707106781186546));
#17308=DIRECTION('ref_axis',(1.,0.,0.));
#17309=DIRECTION('',(1.,0.,0.));
#17310=DIRECTION('center_axis',(0.,0.707106781186549,0.707106781186546));
#17311=DIRECTION('ref_axis',(1.,0.,0.));
#17312=DIRECTION('',(1.,0.,0.));
#17313=DIRECTION('center_axis',(0.707106781186545,0.70710678118655,0.));
#17314=DIRECTION('ref_axis',(0.,0.,-1.));
#17315=DIRECTION('',(0.,0.,-1.));
#17316=DIRECTION('',(0.577350269189628,-0.577350269189624,0.577350269189626));
#17317=DIRECTION('center_axis',(0.,0.707106781186549,0.707106781186546));
#17318=DIRECTION('ref_axis',(1.,0.,0.));
#17319=DIRECTION('',(1.,0.,0.));
#17320=DIRECTION('center_axis',(0.,-1.,0.));
#17321=DIRECTION('ref_axis',(1.,0.,0.));
#17322=DIRECTION('',(0.,0.,1.));
#17323=DIRECTION('center_axis',(0.,0.,1.));
#17324=DIRECTION('ref_axis',(-0.707106781186549,-0.707106781186546,0.));
#17325=DIRECTION('',(0.,0.,-1.));
#17326=DIRECTION('center_axis',(-1.,0.,0.));
#17327=DIRECTION('ref_axis',(0.,-1.,0.));
#17328=DIRECTION('',(0.,0.,1.));
#17329=DIRECTION('center_axis',(0.,0.,1.));
#17330=DIRECTION('ref_axis',(-0.707106781186547,0.707106781186548,0.));
#17331=DIRECTION('center_axis',(1.,0.,0.));
#17332=DIRECTION('ref_axis',(0.,1.,0.));
#17333=DIRECTION('',(0.,-1.,0.));
#17334=DIRECTION('center_axis',(0.,0.,1.));
#17335=DIRECTION('ref_axis',(1.,0.,0.));
#17336=DIRECTION('center_axis',(0.,0.,1.));
#17337=DIRECTION('ref_axis',(1.,0.,0.));
#17338=DIRECTION('',(0.,-1.,0.));
#17339=DIRECTION('center_axis',(1.,0.,0.));
#17340=DIRECTION('ref_axis',(0.,1.,0.));
#17341=DIRECTION('center_axis',(0.,0.,1.));
#17342=DIRECTION('ref_axis',(1.,0.,0.));
#17343=DIRECTION('',(0.730513754696385,0.650233639534332,0.208676467809204));
#17344=DIRECTION('',(-0.730513754696388,-0.650233639534325,0.208676467809214));
#17345=DIRECTION('center_axis',(0.,1.,0.));
#17346=DIRECTION('ref_axis',(-1.,0.,0.));
#17347=DIRECTION('',(-0.491046375823994,-0.70710678118655,-0.508796085667056));
#17348=DIRECTION('center_axis',(0.,-1.,0.));
#17349=DIRECTION('ref_axis',(-1.,0.,0.));
#17350=DIRECTION('center_axis',(0.,-1.,0.));
#17351=DIRECTION('ref_axis',(-1.,0.,0.));
#17352=DIRECTION('',(0.491046375823994,0.70710678118655,-0.508796085667056));
#17353=DIRECTION('center_axis',(0.,-1.,0.));
#17354=DIRECTION('ref_axis',(1.,0.,0.));
#17355=DIRECTION('',(0.,-1.,0.));
#17356=DIRECTION('center_axis',(0.,-1.,0.));
#17357=DIRECTION('ref_axis',(1.,0.,0.));
#17358=DIRECTION('',(-0.730513754696398,0.650233639534323,-0.208676467809188));
#17359=DIRECTION('',(0.730513754696391,-0.650233639534327,-0.208676467809201));
#17360=DIRECTION('center_axis',(0.,1.,0.));
#17361=DIRECTION('ref_axis',(1.,0.,0.));
#17362=DIRECTION('',(0.491046375823994,-0.70710678118655,0.508796085667056));
#17363=DIRECTION('center_axis',(0.,-1.,0.));
#17364=DIRECTION('ref_axis',(1.,0.,0.));
#17365=DIRECTION('',(-0.491046375823994,0.70710678118655,0.508796085667056));
#17366=DIRECTION('center_axis',(0.,-1.,0.));
#17367=DIRECTION('ref_axis',(1.,0.,0.));
#17368=DIRECTION('',(0.,-1.,0.));
#17369=DIRECTION('center_axis',(0.,-1.,0.));
#17370=DIRECTION('ref_axis',(1.,0.,0.));
#17371=DIRECTION('center_axis',(1.,0.,0.));
#17372=DIRECTION('ref_axis',(0.,0.,-1.));
#17373=DIRECTION('',(-0.707106781186547,8.65956056235493E-17,-0.707106781186547));
#17374=DIRECTION('center_axis',(-1.,0.,0.));
#17375=DIRECTION('ref_axis',(0.,0.,-1.));
#17376=DIRECTION('center_axis',(-1.,0.,0.));
#17377=DIRECTION('ref_axis',(0.,0.,-1.));
#17378=DIRECTION('',(-1.,0.,0.));
#17379=DIRECTION('center_axis',(1.,0.,0.));
#17380=DIRECTION('ref_axis',(0.,0.,-1.));
#17381=DIRECTION('center_axis',(-1.,0.,0.));
#17382=DIRECTION('ref_axis',(0.,0.,-1.));
#17383=DIRECTION('center_axis',(-1.,0.,0.));
#17384=DIRECTION('ref_axis',(0.,0.,-1.));
#17385=DIRECTION('',(0.707106781186547,-8.65956056235493E-17,-0.707106781186547));
#17386=DIRECTION('center_axis',(1.,0.,0.));
#17387=DIRECTION('ref_axis',(0.,0.,1.));
#17388=DIRECTION('',(0.,0.,1.));
#17389=DIRECTION('',(0.,-1.,0.));
#17390=DIRECTION('center_axis',(0.,1.,0.));
#17391=DIRECTION('ref_axis',(1.,0.,0.));
#17392=DIRECTION('center_axis',(0.,1.,0.));
#17393=DIRECTION('ref_axis',(1.,0.,0.));
#17394=DIRECTION('center_axis',(0.,-0.5,0.866025403784439));
#17395=DIRECTION('ref_axis',(0.,0.866025403784439,0.5));
#17396=DIRECTION('',(-1.,0.,0.));
#17397=DIRECTION('center_axis',(0.,-1.,-1.354199074918E-16));
#17398=DIRECTION('ref_axis',(0.,-1.354199074918E-16,1.));
#17399=DIRECTION('',(-1.,0.,0.));
#17400=DIRECTION('center_axis',(0.,-0.499999999999999,-0.866025403784439));
#17401=DIRECTION('ref_axis',(0.,-0.866025403784439,0.499999999999999));
#17402=DIRECTION('center_axis',(0.,-0.499999999999999,-0.866025403784439));
#17403=DIRECTION('ref_axis',(0.,0.866025403784439,-0.499999999999999));
#17404=DIRECTION('',(1.,0.,0.));
#17405=DIRECTION('center_axis',(0.,-1.,-1.354199074918E-16));
#17406=DIRECTION('ref_axis',(0.,1.354199074918E-16,-1.));
#17407=DIRECTION('',(1.,0.,0.));
#17408=DIRECTION('center_axis',(0.,-0.5,0.866025403784439));
#17409=DIRECTION('ref_axis',(0.,-0.866025403784439,-0.5));
#17410=DIRECTION('center_axis',(0.,0.,1.));
#17411=DIRECTION('ref_axis',(-1.,0.,0.));
#17412=DIRECTION('',(-1.,0.,0.));
#17413=DIRECTION('center_axis',(0.,-1.,0.));
#17414=DIRECTION('ref_axis',(0.,0.,-1.));
#17415=DIRECTION('center_axis',(0.,0.,1.));
#17416=DIRECTION('ref_axis',(1.,0.,0.));
#20523=CARTESIAN_POINT('',(0.,0.,0.));
#20524=CARTESIAN_POINT('Origin',(29.95,5.75,-36.75));
#20525=CARTESIAN_POINT('',(30.2,5.5,-40.));
#20526=CARTESIAN_POINT('',(29.7,6.,-40.));
#20527=CARTESIAN_POINT('',(25.275,10.425,-40.));
#20528=CARTESIAN_POINT('',(29.7,6.,-33.));
#20529=CARTESIAN_POINT('',(29.7,6.,-36.75));
#20530=CARTESIAN_POINT('',(30.2,5.5,-33.));
#20531=CARTESIAN_POINT('',(29.7,6.,-33.));
#20532=CARTESIAN_POINT('',(30.2,5.5,-36.75));
#20533=CARTESIAN_POINT('Origin',(29.95,5.55111512312578E-16,-33.));
#20534=CARTESIAN_POINT('',(29.7,-6.,-33.));
#20535=CARTESIAN_POINT('',(30.2,-5.5,-33.));
#20536=CARTESIAN_POINT('',(29.7,-6.,-33.));
#20537=CARTESIAN_POINT('Origin',(30.2,5.55111512312578E-16,-33.));
#20538=CARTESIAN_POINT('Origin',(29.7,5.55111512312578E-16,-33.));
#20539=CARTESIAN_POINT('Origin',(29.95,-5.75,-33.25));
#20540=CARTESIAN_POINT('',(29.7,-6.,-40.));
#20541=CARTESIAN_POINT('',(30.2,-5.5,-40.));
#20542=CARTESIAN_POINT('',(24.525,-11.175,-40.));
#20543=CARTESIAN_POINT('',(30.2,-5.5,-33.25));
#20544=CARTESIAN_POINT('',(29.7,-6.,-33.25));
#20545=CARTESIAN_POINT('Origin',(25.2,-6.,-33.));
#20546=CARTESIAN_POINT('',(25.7,-6.,-33.));
#20547=CARTESIAN_POINT('',(25.2,-6.,-33.));
#20548=CARTESIAN_POINT('',(25.7,-6.,-40.));
#20549=CARTESIAN_POINT('',(25.7,-6.,-33.25));
#20550=CARTESIAN_POINT('',(14.6,-6.,-40.));
#20551=CARTESIAN_POINT('Origin',(25.2,5.55111512312578E-16,-33.));
#20552=CARTESIAN_POINT('',(25.7,6.,-33.));
#20553=CARTESIAN_POINT('',(25.2,6.,-33.));
#20554=CARTESIAN_POINT('Origin',(25.7,5.55111512312578E-16,-33.));
#20555=CARTESIAN_POINT('Origin',(25.2,6.,-40.));
#20556=CARTESIAN_POINT('',(25.7,6.,-40.));
#20557=CARTESIAN_POINT('',(14.6,6.,-40.));
#20558=CARTESIAN_POINT('',(25.7,6.,-36.75));
#20559=CARTESIAN_POINT('Origin',(25.45,5.75,-36.75));
#20560=CARTESIAN_POINT('',(25.2,5.5,-40.));
#20561=CARTESIAN_POINT('',(18.275,-1.42500000000001,-40.));
#20562=CARTESIAN_POINT('',(25.2,5.5,-33.));
#20563=CARTESIAN_POINT('',(25.2,5.5,-36.75));
#20564=CARTESIAN_POINT('',(25.2,5.5,-33.));
#20565=CARTESIAN_POINT('Origin',(25.45,5.55111512312578E-16,-33.));
#20566=CARTESIAN_POINT('',(25.2,-5.5,-33.));
#20567=CARTESIAN_POINT('',(25.2,-5.5,-33.));
#20568=CARTESIAN_POINT('Origin',(25.2,5.55111512312578E-16,-33.));
#20569=CARTESIAN_POINT('Origin',(25.45,-5.75,-33.25));
#20570=CARTESIAN_POINT('',(25.2,-5.5,-40.));
#20571=CARTESIAN_POINT('',(19.025,0.675000000000006,-40.));
#20572=CARTESIAN_POINT('',(25.2,-5.5,-33.25));
#20573=CARTESIAN_POINT('Origin',(25.2,0.,-33.5));
#20574=CARTESIAN_POINT('',(25.2,-0.75,-40.));
#20575=CARTESIAN_POINT('',(25.2,4.05,-35.338268590218));
#20576=CARTESIAN_POINT('',(25.2,2.77555756156289E-15,-37.676537180436));
#20577=CARTESIAN_POINT('',(25.2,1.02924682452695,-37.0823012492328));
#20578=CARTESIAN_POINT('',(25.2,4.05,-30.661731409782));
#20579=CARTESIAN_POINT('',(25.2,4.05,-34.2747967278116));
#20580=CARTESIAN_POINT('',(25.2,5.55111512312578E-16,-28.323462819564));
#20581=CARTESIAN_POINT('',(25.2,3.02075317547306,-30.0674954785788));
#20582=CARTESIAN_POINT('',(25.2,-4.05,-30.661731409782));
#20583=CARTESIAN_POINT('',(25.2,-1.24575317547306,-29.0426987507672));
#20584=CARTESIAN_POINT('',(25.2,-4.05,-35.338268590218));
#20585=CARTESIAN_POINT('',(25.2,-4.05,-32.2252032721884));
#20586=CARTESIAN_POINT('',(25.2,-2.80424682452695,-36.0575045214212));
#20587=CARTESIAN_POINT('Origin',(-29.95,-5.75,-36.75));
#20588=CARTESIAN_POINT('',(-30.2,-5.5,-40.));
#20589=CARTESIAN_POINT('',(-29.7,-6.,-40.));
#20590=CARTESIAN_POINT('',(-22.525,-13.175,-40.));
#20591=CARTESIAN_POINT('',(-29.7,-6.,-33.));
#20592=CARTESIAN_POINT('',(-29.7,-6.,-36.75));
#20593=CARTESIAN_POINT('',(-30.2,-5.5,-33.));
#20594=CARTESIAN_POINT('',(-29.7,-6.,-33.));
#20595=CARTESIAN_POINT('',(-30.2,-5.5,-36.75));
#20596=CARTESIAN_POINT('Origin',(-29.95,5.55111512312578E-16,-33.));
#20597=CARTESIAN_POINT('',(-29.7,6.,-33.));
#20598=CARTESIAN_POINT('',(-30.2,5.5,-33.));
#20599=CARTESIAN_POINT('',(-29.7,6.,-33.));
#20600=CARTESIAN_POINT('Origin',(-30.2,5.55111512312578E-16,-33.));
#20601=CARTESIAN_POINT('Origin',(-29.7,5.55111512312578E-16,-33.));
#20602=CARTESIAN_POINT('Origin',(-29.95,5.75,-33.25));
#20603=CARTESIAN_POINT('',(-29.7,6.,-40.));
#20604=CARTESIAN_POINT('',(-30.2,5.5,-40.));
#20605=CARTESIAN_POINT('',(-23.275,12.425,-40.));
#20606=CARTESIAN_POINT('',(-30.2,5.5,-33.25));
#20607=CARTESIAN_POINT('',(-29.7,6.,-33.25));
#20608=CARTESIAN_POINT('Origin',(-25.2,6.,-33.));
#20609=CARTESIAN_POINT('',(-25.7,6.,-33.));
#20610=CARTESIAN_POINT('',(-25.2,6.,-33.));
#20611=CARTESIAN_POINT('',(-25.7,6.,-40.));
#20612=CARTESIAN_POINT('',(-25.7,6.,-33.25));
#20613=CARTESIAN_POINT('',(-10.6,6.,-40.));
#20614=CARTESIAN_POINT('Origin',(-25.2,5.55111512312578E-16,-33.));
#20615=CARTESIAN_POINT('',(-25.7,-6.,-33.));
#20616=CARTESIAN_POINT('',(-25.2,-6.,-33.));
#20617=CARTESIAN_POINT('Origin',(-25.7,5.55111512312578E-16,-33.));
#20618=CARTESIAN_POINT('Origin',(-25.2,-6.,-40.));
#20619=CARTESIAN_POINT('',(-25.7,-6.,-40.));
#20620=CARTESIAN_POINT('',(-10.6,-6.,-40.));
#20621=CARTESIAN_POINT('',(-25.7,-6.,-36.75));
#20622=CARTESIAN_POINT('Origin',(22.,2.5,-38.));
#20623=CARTESIAN_POINT('',(21.5,2.,-38.));
#20624=CARTESIAN_POINT('',(21.5,2.5,-37.5));
#20625=CARTESIAN_POINT('',(21.5,2.,-38.));
#20626=CARTESIAN_POINT('',(22.,2.5,-38.));
#20627=CARTESIAN_POINT('',(22.,2.5,-38.));
#20628=CARTESIAN_POINT('',(21.5,2.5,-37.5));
#20629=CARTESIAN_POINT('Origin',(21.75,2.25,-40.));
#20630=CARTESIAN_POINT('',(21.5,2.,-40.));
#20631=CARTESIAN_POINT('',(22.,2.5,-40.));
#20632=CARTESIAN_POINT('',(16.375,-3.12500000000001,-40.));
#20633=CARTESIAN_POINT('',(22.,2.5,-40.));
#20634=CARTESIAN_POINT('',(21.5,2.,-40.));
#20635=CARTESIAN_POINT('Origin',(21.75,3.5,-37.75));
#20636=CARTESIAN_POINT('',(21.75,7.75,-37.75));
#20637=CARTESIAN_POINT('',(21.5,7.5,-37.5));
#20638=CARTESIAN_POINT('',(22.6666666666667,8.66666666666666,-38.6666666666667));
#20639=CARTESIAN_POINT('',(21.5,3.5,-37.5));
#20640=CARTESIAN_POINT('',(22.,7.5,-38.));
#20641=CARTESIAN_POINT('',(22.,3.5,-38.));
#20642=CARTESIAN_POINT('',(24.0833333333333,5.41666666666666,-40.0833333333333));
#20643=CARTESIAN_POINT('Origin',(16.,2.25,-37.75));
#20644=CARTESIAN_POINT('',(14.25,2.25,-37.75));
#20645=CARTESIAN_POINT('',(14.5,2.,-38.));
#20646=CARTESIAN_POINT('',(14.9166666666667,1.58333333333333,-38.4166666666667));
#20647=CARTESIAN_POINT('',(16.,2.,-38.));
#20648=CARTESIAN_POINT('',(14.5,2.5,-37.5));
#20649=CARTESIAN_POINT('',(16.,2.5,-37.5));
#20650=CARTESIAN_POINT('',(15.25,3.25,-36.75));
#20651=CARTESIAN_POINT('Origin',(22.,2.,-40.));
#20652=CARTESIAN_POINT('',(22.,7.5,-40.));
#20653=CARTESIAN_POINT('',(22.,0.25,-40.));
#20654=CARTESIAN_POINT('',(22.,7.5,-47.5));
#20655=CARTESIAN_POINT('Origin',(14.,2.,-40.));
#20656=CARTESIAN_POINT('',(14.5,2.,-40.));
#20657=CARTESIAN_POINT('',(14.5,2.,-40.));
#20658=CARTESIAN_POINT('',(9.,2.,-40.));
#20659=CARTESIAN_POINT('Origin',(14.25,2.25,-40.));
#20660=CARTESIAN_POINT('',(14.,2.5,-38.));
#20661=CARTESIAN_POINT('',(14.5,2.,-37.5));
#20662=CARTESIAN_POINT('',(14.,2.5,-40.));
#20663=CARTESIAN_POINT('',(14.,2.5,-40.));
#20664=CARTESIAN_POINT('',(12.625,3.875,-40.));
#20665=CARTESIAN_POINT('Origin',(29.95,0.,-33.));
#20666=CARTESIAN_POINT('',(30.2,-3.24531401774048E-16,-30.35));
#20667=CARTESIAN_POINT('Origin',(30.2,0.,-33.));
#20668=CARTESIAN_POINT('',(29.7,2.63299061816681E-16,-30.85));
#20669=CARTESIAN_POINT('',(29.95,-2.93915231795365E-16,-30.6));
#20670=CARTESIAN_POINT('Origin',(29.7,0.,-33.));
#20671=CARTESIAN_POINT('Origin',(30.2,0.,-33.));
#20672=CARTESIAN_POINT('',(28.9,-2.63299061816681E-16,-30.85));
#20673=CARTESIAN_POINT('',(30.2,2.63299061816681E-16,-30.85));
#20674=CARTESIAN_POINT('Origin',(28.9,0.,-33.));
#20675=CARTESIAN_POINT('Origin',(30.2,0.,-33.5));
#20676=CARTESIAN_POINT('',(30.2,-0.75,-40.));
#20677=CARTESIAN_POINT('Origin',(-29.95,0.,-33.));
#20678=CARTESIAN_POINT('',(-30.2,3.24531401774048E-16,-30.35));
#20679=CARTESIAN_POINT('Origin',(-30.2,0.,-33.));
#20680=CARTESIAN_POINT('',(-29.7,-2.63299061816681E-16,-30.85));
#20681=CARTESIAN_POINT('',(-29.95,2.93915231795365E-16,-30.6));
#20682=CARTESIAN_POINT('Origin',(-29.7,0.,-33.));
#20683=CARTESIAN_POINT('Origin',(-30.2,0.,-33.));
#20684=CARTESIAN_POINT('',(-28.9,2.63299061816681E-16,-30.85));
#20685=CARTESIAN_POINT('',(-30.2,-2.63299061816681E-16,-30.85));
#20686=CARTESIAN_POINT('Origin',(-28.9,0.,-33.));
#20687=CARTESIAN_POINT('Origin',(-30.2,0.,-33.5));
#20688=CARTESIAN_POINT('',(-30.2,-0.75,-40.));
#20689=CARTESIAN_POINT('Origin',(28.65,0.,-33.));
#20690=CARTESIAN_POINT('',(28.4,3.24531401774048E-16,-30.35));
#20691=CARTESIAN_POINT('',(28.65,-2.93915231795365E-16,-30.6));
#20692=CARTESIAN_POINT('Origin',(28.4,0.,-33.));
#20693=CARTESIAN_POINT('Origin',(28.4,0.,-33.));
#20694=CARTESIAN_POINT('',(28.4,3.55,-35.0495934556232));
#20695=CARTESIAN_POINT('',(28.4,3.55,-30.9504065443768));
#20696=CARTESIAN_POINT('',(28.4,3.55,-35.0495934556232));
#20697=CARTESIAN_POINT('',(28.4,-5.55111512312578E-16,-37.0991869112463));
#20698=CARTESIAN_POINT('',(28.4,-7.53008419494684E-16,-37.0991869112463));
#20699=CARTESIAN_POINT('',(28.4,-3.55,-35.0495934556232));
#20700=CARTESIAN_POINT('',(28.4,-3.55,-35.0495934556232));
#20701=CARTESIAN_POINT('',(28.4,-3.55,-30.9504065443768));
#20702=CARTESIAN_POINT('',(28.4,-3.55,-30.9504065443768));
#20703=CARTESIAN_POINT('',(28.4,0.,-28.9008130887537));
#20704=CARTESIAN_POINT('',(28.4,2.51002806498228E-16,-28.9008130887537));
#20705=CARTESIAN_POINT('',(28.4,3.55,-30.9504065443768));
#20706=CARTESIAN_POINT('Origin',(25.45,-1.12075317547306,-29.2592051017133));
#20707=CARTESIAN_POINT('',(25.7,2.51002806498228E-16,-28.9008130887537));
#20708=CARTESIAN_POINT('',(25.2,5.55111512312578E-16,-28.323462819564));
#20709=CARTESIAN_POINT('',(25.7,-3.55,-30.9504065443768));
#20710=CARTESIAN_POINT('',(25.7,-0.995753175473055,-29.4757114526594));
#20711=CARTESIAN_POINT('',(25.2,-4.05,-30.661731409782));
#20712=CARTESIAN_POINT('Origin',(25.45,2.89575317547306,-30.2840018295249));
#20713=CARTESIAN_POINT('',(25.7,3.55,-30.9504065443768));
#20714=CARTESIAN_POINT('',(25.2,4.05,-30.661731409782));
#20715=CARTESIAN_POINT('',(25.7,2.77075317547306,-30.500508180471));
#20716=CARTESIAN_POINT('Origin',(25.45,0.904246824526946,-36.8657948982867));
#20717=CARTESIAN_POINT('',(25.7,-7.53008419494684E-16,-37.0991869112463));
#20718=CARTESIAN_POINT('',(25.2,2.77555756156289E-15,-37.676537180436));
#20719=CARTESIAN_POINT('',(25.7,3.55,-35.0495934556232));
#20720=CARTESIAN_POINT('',(25.7,0.779246824526944,-36.6492885473405));
#20721=CARTESIAN_POINT('',(25.7,3.55,-35.0495934556232));
#20722=CARTESIAN_POINT('Origin',(25.45,-2.67924682452694,-35.8409981704751));
#20723=CARTESIAN_POINT('',(25.7,-3.55,-35.0495934556232));
#20724=CARTESIAN_POINT('',(25.7,-2.55424682452694,-35.624491819529));
#20725=CARTESIAN_POINT('',(25.2,-4.05,-35.338268590218));
#20726=CARTESIAN_POINT('Origin',(25.45,3.8,-34.2747967278116));
#20727=CARTESIAN_POINT('',(25.7,3.55,-34.2747967278116));
#20728=CARTESIAN_POINT('Origin',(25.45,-3.8,-32.2252032721884));
#20729=CARTESIAN_POINT('',(25.7,-3.55,-32.2252032721884));
#20730=CARTESIAN_POINT('Origin',(25.2,3.55,-30.9504065443768));
#20731=CARTESIAN_POINT('',(25.2,3.55,-30.9504065443768));
#20732=CARTESIAN_POINT('',(25.2,2.51002806498228E-16,-28.9008130887537));
#20733=CARTESIAN_POINT('Origin',(25.2,3.55,-35.0495934556232));
#20734=CARTESIAN_POINT('',(25.2,3.55,-35.0495934556232));
#20735=CARTESIAN_POINT('Origin',(25.2,-7.53008419494684E-16,-37.0991869112463));
#20736=CARTESIAN_POINT('',(25.2,-7.53008419494684E-16,-37.0991869112463));
#20737=CARTESIAN_POINT('Origin',(-28.65,0.,-33.));
#20738=CARTESIAN_POINT('',(-28.4,-3.24531401774048E-16,-30.35));
#20739=CARTESIAN_POINT('',(-28.65,2.93915231795365E-16,-30.6));
#20740=CARTESIAN_POINT('Origin',(-28.4,0.,-33.));
#20741=CARTESIAN_POINT('Origin',(-28.4,0.,-33.));
#20742=CARTESIAN_POINT('',(-28.4,3.55,-30.9504065443768));
#20743=CARTESIAN_POINT('',(-28.4,3.55,-35.0495934556232));
#20744=CARTESIAN_POINT('',(-28.4,3.55,-35.0495934556232));
#20745=CARTESIAN_POINT('',(-28.4,0.,-28.9008130887537));
#20746=CARTESIAN_POINT('',(-28.4,3.55,-30.9504065443768));
#20747=CARTESIAN_POINT('',(-28.4,-3.55,-30.9504065443768));
#20748=CARTESIAN_POINT('',(-28.4,2.51002806498228E-16,-28.9008130887537));
#20749=CARTESIAN_POINT('',(-28.4,-3.55,-35.0495934556232));
#20750=CARTESIAN_POINT('',(-28.4,-3.55,-30.9504065443768));
#20751=CARTESIAN_POINT('',(-28.4,-5.55111512312578E-16,-37.0991869112463));
#20752=CARTESIAN_POINT('',(-28.4,-3.55,-35.0495934556232));
#20753=CARTESIAN_POINT('',(-28.4,-7.53008419494684E-16,-37.0991869112463));
#20754=CARTESIAN_POINT('Origin',(-25.45,5.75,-33.25));
#20755=CARTESIAN_POINT('',(-25.2,5.5,-40.));
#20756=CARTESIAN_POINT('',(-16.275,-3.42500000000001,-40.));
#20757=CARTESIAN_POINT('',(-25.2,5.5,-33.));
#20758=CARTESIAN_POINT('',(-25.7,6.,-33.));
#20759=CARTESIAN_POINT('',(-25.2,5.5,-33.25));
#20760=CARTESIAN_POINT('Origin',(-25.45,5.55111512312578E-16,-33.));
#20761=CARTESIAN_POINT('',(-25.2,-5.5,-33.));
#20762=CARTESIAN_POINT('',(-25.7,-6.,-33.));
#20763=CARTESIAN_POINT('Origin',(-25.2,5.55111512312578E-16,-33.));
#20764=CARTESIAN_POINT('Origin',(-25.45,-5.75,-36.75));
#20765=CARTESIAN_POINT('',(-25.2,-5.5,-40.));
#20766=CARTESIAN_POINT('',(-17.025,2.675,-40.));
#20767=CARTESIAN_POINT('',(-25.2,-5.5,-36.75));
#20768=CARTESIAN_POINT('Origin',(-25.45,-0.904246824526945,-36.8657948982867));
#20769=CARTESIAN_POINT('',(-25.2,-4.05,-35.338268590218));
#20770=CARTESIAN_POINT('',(-25.2,2.22044604925031E-15,-37.676537180436));
#20771=CARTESIAN_POINT('',(-25.2,-1.02924682452694,-37.0823012492328));
#20772=CARTESIAN_POINT('',(-25.7,-7.53008419494684E-16,-37.0991869112463));
#20773=CARTESIAN_POINT('',(-25.2,2.22044604925031E-15,-37.676537180436));
#20774=CARTESIAN_POINT('',(-25.7,-3.55,-35.0495934556232));
#20775=CARTESIAN_POINT('',(-25.7,-0.779246824526944,-36.6492885473405));
#20776=CARTESIAN_POINT('',(-25.2,-4.05,-35.338268590218));
#20777=CARTESIAN_POINT('Origin',(-25.45,2.67924682452694,-35.8409981704751));
#20778=CARTESIAN_POINT('',(-25.2,4.05,-35.338268590218));
#20779=CARTESIAN_POINT('',(-25.2,2.80424682452694,-36.0575045214212));
#20780=CARTESIAN_POINT('',(-25.7,3.55,-35.0495934556232));
#20781=CARTESIAN_POINT('',(-25.2,4.05,-35.338268590218));
#20782=CARTESIAN_POINT('',(-25.7,2.55424682452694,-35.624491819529));
#20783=CARTESIAN_POINT('Origin',(-25.45,1.12075317547306,-29.2592051017133));
#20784=CARTESIAN_POINT('',(-25.2,4.05,-30.661731409782));
#20785=CARTESIAN_POINT('',(-25.2,0.,-28.323462819564));
#20786=CARTESIAN_POINT('',(-25.2,1.24575317547306,-29.0426987507672));
#20787=CARTESIAN_POINT('',(-25.7,2.51002806498228E-16,-28.9008130887537));
#20788=CARTESIAN_POINT('',(-25.2,0.,-28.323462819564));
#20789=CARTESIAN_POINT('',(-25.7,3.55,-30.9504065443768));
#20790=CARTESIAN_POINT('',(-25.7,0.995753175473055,-29.4757114526594));
#20791=CARTESIAN_POINT('',(-25.7,3.55,-30.9504065443768));
#20792=CARTESIAN_POINT('Origin',(-25.45,-2.89575317547306,-30.2840018295249));
#20793=CARTESIAN_POINT('',(-25.7,-3.55,-30.9504065443768));
#20794=CARTESIAN_POINT('',(-25.7,-2.77075317547306,-30.500508180471));
#20795=CARTESIAN_POINT('',(-25.2,-4.05,-30.661731409782));
#20796=CARTESIAN_POINT('',(-25.2,-3.02075317547306,-30.0674954785788));
#20797=CARTESIAN_POINT('',(-25.2,-4.05,-30.661731409782));
#20798=CARTESIAN_POINT('Origin',(-25.45,3.8,-32.2252032721884));
#20799=CARTESIAN_POINT('',(-25.2,4.05,-32.2252032721884));
#20800=CARTESIAN_POINT('',(-25.7,3.55,-32.2252032721884));
#20801=CARTESIAN_POINT('Origin',(-25.45,-3.8,-34.2747967278116));
#20802=CARTESIAN_POINT('',(-25.7,-3.55,-34.2747967278116));
#20803=CARTESIAN_POINT('',(-25.2,-4.05,-34.2747967278116));
#20804=CARTESIAN_POINT('Origin',(-25.2,3.55,-35.0495934556232));
#20805=CARTESIAN_POINT('',(-25.2,3.55,-35.0495934556232));
#20806=CARTESIAN_POINT('',(-25.2,-7.53008419494684E-16,-37.0991869112463));
#20807=CARTESIAN_POINT('Origin',(-25.2,3.55,-30.9504065443768));
#20808=CARTESIAN_POINT('',(-25.2,3.55,-30.9504065443768));
#20809=CARTESIAN_POINT('Origin',(-25.2,0.,-28.9008130887537));
#20810=CARTESIAN_POINT('',(-25.2,2.51002806498228E-16,-28.9008130887537));
#20811=CARTESIAN_POINT('Origin',(-25.2,0.,-33.5));
#20812=CARTESIAN_POINT('',(-25.2,-0.75,-40.));
#20813=CARTESIAN_POINT('Origin',(-23.5,2.,-38.));
#20814=CARTESIAN_POINT('',(-24.,2.5,-38.));
#20815=CARTESIAN_POINT('',(-23.5,2.5,-37.5));
#20816=CARTESIAN_POINT('',(-24.,2.5,-38.));
#20817=CARTESIAN_POINT('',(-23.5,2.,-38.));
#20818=CARTESIAN_POINT('',(-23.5,2.,-38.));
#20819=CARTESIAN_POINT('',(-23.5,2.5,-37.5));
#20820=CARTESIAN_POINT('Origin',(-23.75,2.25,-40.));
#20821=CARTESIAN_POINT('',(-24.,2.5,-40.));
#20822=CARTESIAN_POINT('',(-23.5,2.,-40.));
#20823=CARTESIAN_POINT('',(-15.875,-5.625,-40.));
#20824=CARTESIAN_POINT('',(-23.5,2.,-40.));
#20825=CARTESIAN_POINT('',(-24.,2.5,-40.));
#20826=CARTESIAN_POINT('Origin',(-16.,2.5,-38.));
#20827=CARTESIAN_POINT('',(-16.5,2.,-38.));
#20828=CARTESIAN_POINT('',(-16.5,2.5,-37.5));
#20829=CARTESIAN_POINT('',(-16.5,2.,-38.));
#20830=CARTESIAN_POINT('',(-16.,2.5,-38.));
#20831=CARTESIAN_POINT('',(-16.,2.5,-38.));
#20832=CARTESIAN_POINT('',(-16.5,2.5,-37.5));
#20833=CARTESIAN_POINT('Origin',(-16.25,2.25,-40.));
#20834=CARTESIAN_POINT('',(-16.5,2.,-40.));
#20835=CARTESIAN_POINT('',(-16.,2.5,-40.));
#20836=CARTESIAN_POINT('',(-12.125,6.375,-40.));
#20837=CARTESIAN_POINT('',(-16.,2.5,-40.));
#20838=CARTESIAN_POINT('',(-16.5,2.,-40.));
#20839=CARTESIAN_POINT('Origin',(-16.25,3.5,-37.75));
#20840=CARTESIAN_POINT('',(-16.25,7.75,-37.75));
#20841=CARTESIAN_POINT('',(-16.5,7.5,-37.5));
#20842=CARTESIAN_POINT('',(-12.1666666666666,11.8333333333333,-41.8333333333334));
#20843=CARTESIAN_POINT('',(-16.5,3.5,-37.5));
#20844=CARTESIAN_POINT('',(-16.,7.5,-38.));
#20845=CARTESIAN_POINT('',(-16.,3.5,-38.));
#20846=CARTESIAN_POINT('',(-13.9166666666667,5.41666666666667,-40.0833333333333));
#20847=CARTESIAN_POINT('Origin',(-22.,2.25,-37.75));
#20848=CARTESIAN_POINT('',(-22.,2.5,-37.5));
#20849=CARTESIAN_POINT('',(-22.,2.,-38.));
#20850=CARTESIAN_POINT('Origin',(-23.75,6.5,-37.75));
#20851=CARTESIAN_POINT('',(-23.75,7.75,-37.75));
#20852=CARTESIAN_POINT('',(-24.,7.5,-38.));
#20853=CARTESIAN_POINT('',(-25.5833333333333,5.91666666666667,-39.5833333333333));
#20854=CARTESIAN_POINT('',(-24.,6.5,-38.));
#20855=CARTESIAN_POINT('',(-23.5,7.5,-37.5));
#20856=CARTESIAN_POINT('',(-23.5,6.5,-37.5));
#20857=CARTESIAN_POINT('',(-17.5,1.50000000000001,-31.5));
#20858=CARTESIAN_POINT('Origin',(-24.,2.,-40.));
#20859=CARTESIAN_POINT('',(-10.,2.,-40.));
#20860=CARTESIAN_POINT('Origin',(-24.,8.,-40.));
#20861=CARTESIAN_POINT('',(-24.,7.5,-40.));
#20862=CARTESIAN_POINT('',(-24.,7.5,-47.5));
#20863=CARTESIAN_POINT('',(-24.,3.25,-40.));
#20864=CARTESIAN_POINT('Origin',(-23.75,7.75,-47.5));
#20865=CARTESIAN_POINT('',(-23.5,8.,-38.));
#20866=CARTESIAN_POINT('',(-24.,7.5,-37.5));
#20867=CARTESIAN_POINT('',(-23.5,8.,-40.5));
#20868=CARTESIAN_POINT('',(-23.5,8.,-47.5));
#20869=CARTESIAN_POINT('',(-24.,7.5,-40.));
#20870=CARTESIAN_POINT('Origin',(-3.5,2.,-38.));
#20871=CARTESIAN_POINT('',(-4.,2.5,-38.));
#20872=CARTESIAN_POINT('',(-3.5,2.5,-37.5));
#20873=CARTESIAN_POINT('',(-4.,2.5,-38.));
#20874=CARTESIAN_POINT('',(-3.5,2.,-38.));
#20875=CARTESIAN_POINT('',(-3.5,2.,-38.));
#20876=CARTESIAN_POINT('',(-3.5,2.5,-37.5));
#20877=CARTESIAN_POINT('Origin',(-3.75,2.25,-40.));
#20878=CARTESIAN_POINT('',(-4.,2.5,-40.));
#20879=CARTESIAN_POINT('',(-3.5,2.,-40.));
#20880=CARTESIAN_POINT('',(-0.874999999999997,-0.624999999999997,-40.));
#20881=CARTESIAN_POINT('',(-3.5,2.,-40.));
#20882=CARTESIAN_POINT('',(-4.,2.5,-40.));
#20883=CARTESIAN_POINT('Origin',(4.,2.5,-38.));
#20884=CARTESIAN_POINT('',(3.5,2.,-38.));
#20885=CARTESIAN_POINT('',(3.5,2.5,-37.5));
#20886=CARTESIAN_POINT('',(3.5,2.,-38.));
#20887=CARTESIAN_POINT('',(4.,2.5,-38.));
#20888=CARTESIAN_POINT('',(4.,2.5,-38.));
#20889=CARTESIAN_POINT('',(3.5,2.5,-37.5));
#20890=CARTESIAN_POINT('Origin',(3.75,2.25,-40.));
#20891=CARTESIAN_POINT('',(3.5,2.,-40.));
#20892=CARTESIAN_POINT('',(4.,2.5,-40.));
#20893=CARTESIAN_POINT('',(2.875,1.375,-40.));
#20894=CARTESIAN_POINT('',(4.,2.5,-40.));
#20895=CARTESIAN_POINT('',(3.5,2.,-40.));
#20896=CARTESIAN_POINT('Origin',(3.75,3.5,-37.75));
#20897=CARTESIAN_POINT('',(3.75,7.75,-37.75));
#20898=CARTESIAN_POINT('',(3.5,7.5,-37.5));
#20899=CARTESIAN_POINT('',(6.16666666666669,10.1666666666667,-40.1666666666667));
#20900=CARTESIAN_POINT('',(3.5,3.5,-37.5));
#20901=CARTESIAN_POINT('',(4.,7.5,-38.));
#20902=CARTESIAN_POINT('',(4.,3.5,-38.));
#20903=CARTESIAN_POINT('',(6.08333333333334,5.41666666666668,-40.0833333333333));
#20904=CARTESIAN_POINT('Origin',(-2.,2.25,-37.75));
#20905=CARTESIAN_POINT('',(-2.,2.5,-37.5));
#20906=CARTESIAN_POINT('',(-2.,2.,-38.));
#20907=CARTESIAN_POINT('Origin',(-3.75,6.5,-37.75));
#20908=CARTESIAN_POINT('',(-3.75,7.75,-37.75));
#20909=CARTESIAN_POINT('',(-4.,7.5,-38.));
#20910=CARTESIAN_POINT('',(-5.58333333333333,5.91666666666667,-39.5833333333333));
#20911=CARTESIAN_POINT('',(-4.,6.5,-38.));
#20912=CARTESIAN_POINT('',(-3.5,7.5,-37.5));
#20913=CARTESIAN_POINT('',(-3.5,6.5,-37.5));
#20914=CARTESIAN_POINT('',(0.833333333333363,3.16666666666667,-33.1666666666667));
#20915=CARTESIAN_POINT('Origin',(-4.,2.,-40.));
#20916=CARTESIAN_POINT('',(-2.77555756156289E-15,2.,-40.));
#20917=CARTESIAN_POINT('Origin',(-4.,8.,-40.));
#20918=CARTESIAN_POINT('',(-4.,7.5,-40.));
#20919=CARTESIAN_POINT('',(-4.,7.5,-47.5));
#20920=CARTESIAN_POINT('',(-4.,3.25,-40.));
#20921=CARTESIAN_POINT('Origin',(-3.75,7.75,-47.5));
#20922=CARTESIAN_POINT('',(-3.5,8.,-38.));
#20923=CARTESIAN_POINT('',(-4.,7.5,-37.5));
#20924=CARTESIAN_POINT('',(-3.5,8.,-40.5));
#20925=CARTESIAN_POINT('',(-3.5,8.,-47.5));
#20926=CARTESIAN_POINT('',(-4.,7.5,-40.));
#20927=CARTESIAN_POINT('Origin',(14.25,6.5,-37.75));
#20928=CARTESIAN_POINT('',(14.5,7.5,-37.5));
#20929=CARTESIAN_POINT('',(14.5,6.5,-37.5));
#20930=CARTESIAN_POINT('',(14.25,7.75,-37.75));
#20931=CARTESIAN_POINT('',(17.3333333333334,4.66666666666667,-34.6666666666667));
#20932=CARTESIAN_POINT('',(14.,7.5,-38.));
#20933=CARTESIAN_POINT('',(12.4166666666667,5.91666666666667,-39.5833333333333));
#20934=CARTESIAN_POINT('',(14.,6.5,-38.));
#20935=CARTESIAN_POINT('Origin',(14.,8.,-40.));
#20936=CARTESIAN_POINT('',(14.,7.5,-40.));
#20937=CARTESIAN_POINT('',(14.,7.5,-47.5));
#20938=CARTESIAN_POINT('',(14.,3.25,-40.));
#20939=CARTESIAN_POINT('Origin',(14.25,7.75,-47.5));
#20940=CARTESIAN_POINT('',(14.5,8.,-38.));
#20941=CARTESIAN_POINT('',(14.,7.5,-37.5));
#20942=CARTESIAN_POINT('',(14.5,8.,-40.5));
#20943=CARTESIAN_POINT('',(14.5,8.,-47.5));
#20944=CARTESIAN_POINT('',(14.,7.5,-40.));
#20945=CARTESIAN_POINT('Origin',(6.75,7.75,-53.25));
#20946=CARTESIAN_POINT('',(-31.5,7.5,-53.));
#20947=CARTESIAN_POINT('',(39.5,7.5,-53.));
#20948=CARTESIAN_POINT('',(6.75,7.5,-53.));
#20949=CARTESIAN_POINT('',(40.,8.,-53.5));
#20950=CARTESIAN_POINT('',(34.3750000000001,2.37500000000007,-47.875));
#20951=CARTESIAN_POINT('',(-32.,8.,-53.5));
#20952=CARTESIAN_POINT('',(6.75,8.,-53.5));
#20953=CARTESIAN_POINT('',(-32.,8.,-53.5));
#20954=CARTESIAN_POINT('Origin',(-31.75,7.75,-48.5));
#20955=CARTESIAN_POINT('',(-32.,8.,-41.5));
#20956=CARTESIAN_POINT('',(-32.,8.,-48.5));
#20957=CARTESIAN_POINT('',(-31.5,7.5,-42.));
#20958=CARTESIAN_POINT('',(-18.2916666666667,-5.70833333333324,-55.2083333333334));
#20959=CARTESIAN_POINT('',(-31.5,7.5,-48.5));
#20960=CARTESIAN_POINT('Origin',(-31.5,8.,-53.));
#20961=CARTESIAN_POINT('',(-31.5,-9.,-53.));
#20962=CARTESIAN_POINT('',(-31.5,8.,-53.));
#20963=CARTESIAN_POINT('',(39.5,-9.,-53.));
#20964=CARTESIAN_POINT('',(-31.5,-9.,-53.));
#20965=CARTESIAN_POINT('',(39.5,8.,-53.));
#20966=CARTESIAN_POINT('Origin',(-31.5,8.,-42.));
#20967=CARTESIAN_POINT('',(-31.5,-9.,-42.));
#20968=CARTESIAN_POINT('',(-31.5,8.,-42.));
#20969=CARTESIAN_POINT('',(-31.5,-9.,-42.));
#20970=CARTESIAN_POINT('Origin',(39.75,7.75,-54.));
#20971=CARTESIAN_POINT('',(40.,8.,-41.5));
#20972=CARTESIAN_POINT('',(40.,8.,-54.));
#20973=CARTESIAN_POINT('',(39.5,7.5,-42.));
#20974=CARTESIAN_POINT('',(39.5,7.5,-54.));
#20975=CARTESIAN_POINT('',(39.5,7.5,-42.));
#20976=CARTESIAN_POINT('Origin',(42.25,7.75,-41.75));
#20977=CARTESIAN_POINT('',(42.25,7.5,-42.));
#20978=CARTESIAN_POINT('',(42.25,8.,-41.5));
#20979=CARTESIAN_POINT('Origin',(45.,8.,-55.));
#20980=CARTESIAN_POINT('',(-35.5,8.,-54.5));
#20981=CARTESIAN_POINT('',(43.5,8.,-54.5));
#20982=CARTESIAN_POINT('',(24.5,8.,-54.5));
#20983=CARTESIAN_POINT('',(-35.5,8.,-48.7951833846989));
#20984=CARTESIAN_POINT('',(-35.5,8.,-55.));
#20985=CARTESIAN_POINT('',(-35.5,8.,-46.2048166153011));
#20986=CARTESIAN_POINT('Origin',(-34.25,8.,-47.5));
#20987=CARTESIAN_POINT('',(-35.5,8.,-40.5));
#20988=CARTESIAN_POINT('',(-35.5,8.,-55.));
#20989=CARTESIAN_POINT('',(24.5,8.,-40.5));
#20990=CARTESIAN_POINT('',(-16.5,8.,-38.));
#20991=CARTESIAN_POINT('',(12.5,8.,-38.));
#20992=CARTESIAN_POINT('',(-16.5,8.,-40.5));
#20993=CARTESIAN_POINT('',(-16.5,8.,-47.5));
#20994=CARTESIAN_POINT('',(24.5,8.,-40.5));
#20995=CARTESIAN_POINT('',(3.5,8.,-38.));
#20996=CARTESIAN_POINT('',(22.5,8.,-38.));
#20997=CARTESIAN_POINT('',(3.5,8.,-40.5));
#20998=CARTESIAN_POINT('',(3.5,8.,-47.5));
#20999=CARTESIAN_POINT('',(24.5,8.,-40.5));
#21000=CARTESIAN_POINT('',(21.5,8.,-38.));
#21001=CARTESIAN_POINT('',(31.5,8.,-38.));
#21002=CARTESIAN_POINT('',(21.5,8.,-40.5));
#21003=CARTESIAN_POINT('',(21.5,8.,-47.5));
#21004=CARTESIAN_POINT('',(43.5,8.,-40.5));
#21005=CARTESIAN_POINT('',(24.5,8.,-40.5));
#21006=CARTESIAN_POINT('',(43.5,8.,-46.2048166153011));
#21007=CARTESIAN_POINT('',(43.5,8.,-55.));
#21008=CARTESIAN_POINT('',(43.5,8.,-48.7951833846989));
#21009=CARTESIAN_POINT('Origin',(42.25,8.,-47.5));
#21010=CARTESIAN_POINT('',(43.5,8.,-55.));
#21011=CARTESIAN_POINT('Origin',(24.5,7.75,-54.75));
#21012=CARTESIAN_POINT('',(-35.5,7.5,-55.));
#21013=CARTESIAN_POINT('',(-35.5,7.5,-55.));
#21014=CARTESIAN_POINT('',(43.5,7.5,-55.));
#21015=CARTESIAN_POINT('',(43.5,8.,-54.5));
#21016=CARTESIAN_POINT('',(24.5,7.5,-55.));
#21017=CARTESIAN_POINT('Origin',(-35.5,6.5,-54.75));
#21018=CARTESIAN_POINT('',(-36.5,6.5,-55.));
#21019=CARTESIAN_POINT('',(-37.,6.5,-54.5));
#21020=CARTESIAN_POINT('',(-36.5,6.5,-55.));
#21021=CARTESIAN_POINT('Origin',(-35.5,6.5,-54.5));
#21022=CARTESIAN_POINT('Origin',(-35.5,6.5,-55.));
#21023=CARTESIAN_POINT('Origin',(-36.75,3.25,-54.75));
#21024=CARTESIAN_POINT('',(-36.5,-9.5,-55.));
#21025=CARTESIAN_POINT('',(-37.,-9.5,-54.5));
#21026=CARTESIAN_POINT('',(-36.5,-9.5,-55.));
#21027=CARTESIAN_POINT('',(-37.,3.25,-54.5));
#21028=CARTESIAN_POINT('',(-36.5,3.25,-55.));
#21029=CARTESIAN_POINT('Origin',(-35.5,-9.5,-54.75));
#21030=CARTESIAN_POINT('',(-35.5,-10.5,-55.));
#21031=CARTESIAN_POINT('',(-35.5,-11.,-54.5));
#21032=CARTESIAN_POINT('',(-35.5,-10.5,-55.));
#21033=CARTESIAN_POINT('Origin',(-35.5,-9.5,-54.5));
#21034=CARTESIAN_POINT('Origin',(-35.5,-9.5,-55.));
#21035=CARTESIAN_POINT('Origin',(-16.5,-10.75,-54.75));
#21036=CARTESIAN_POINT('',(43.5,-10.5,-55.));
#21037=CARTESIAN_POINT('',(43.5,-11.,-54.5));
#21038=CARTESIAN_POINT('',(43.5,-10.5,-55.));
#21039=CARTESIAN_POINT('',(-16.5,-11.,-54.5));
#21040=CARTESIAN_POINT('',(-16.5,-10.5,-55.));
#21041=CARTESIAN_POINT('Origin',(43.5,-9.5,-54.75));
#21042=CARTESIAN_POINT('',(44.5,-9.5,-55.));
#21043=CARTESIAN_POINT('',(45.,-9.5,-54.5));
#21044=CARTESIAN_POINT('',(44.5,-9.5,-55.));
#21045=CARTESIAN_POINT('Origin',(43.5,-9.5,-54.5));
#21046=CARTESIAN_POINT('Origin',(43.5,-9.5,-55.));
#21047=CARTESIAN_POINT('Origin',(44.75,-6.25,-54.75));
#21048=CARTESIAN_POINT('',(44.5,6.5,-55.));
#21049=CARTESIAN_POINT('',(45.,6.5,-54.5));
#21050=CARTESIAN_POINT('',(44.5,6.5,-55.));
#21051=CARTESIAN_POINT('',(45.,-6.25,-54.5));
#21052=CARTESIAN_POINT('',(44.5,-6.25,-55.));
#21053=CARTESIAN_POINT('Origin',(43.5,6.5,-54.75));
#21054=CARTESIAN_POINT('Origin',(43.5,6.5,-54.5));
#21055=CARTESIAN_POINT('Origin',(43.5,6.5,-55.));
#21056=CARTESIAN_POINT('Origin',(43.5,-9.5,-55.));
#21057=CARTESIAN_POINT('',(45.,-9.5,-40.5));
#21058=CARTESIAN_POINT('',(45.,-9.5,-55.));
#21059=CARTESIAN_POINT('',(43.5,-11.,-40.5));
#21060=CARTESIAN_POINT('Origin',(43.5,-9.5,-40.5));
#21061=CARTESIAN_POINT('',(43.5,-11.,-55.));
#21062=CARTESIAN_POINT('Origin',(45.,-11.,-55.));
#21063=CARTESIAN_POINT('',(45.,6.5,-40.5));
#21064=CARTESIAN_POINT('',(45.,6.5,-55.));
#21065=CARTESIAN_POINT('',(45.,-6.25,-40.5));
#21066=CARTESIAN_POINT('',(45.,-3.,-44.5));
#21067=CARTESIAN_POINT('Origin',(45.,-3.,-47.5));
#21068=CARTESIAN_POINT('Origin',(43.5,6.5,-55.));
#21069=CARTESIAN_POINT('',(43.9750046174461,7.92280378598205,-47.9927598805759));
#21070=CARTESIAN_POINT('Ctrl Pts',(43.9750046174461,7.92280378598205,-47.9927598805759));
#21071=CARTESIAN_POINT('Ctrl Pts',(43.8929060558365,7.95021248156921,-48.295755755381));
#21072=CARTESIAN_POINT('Ctrl Pts',(43.7266147755088,8.,-48.5764742252605));
#21073=CARTESIAN_POINT('Ctrl Pts',(43.5,8.,-48.7951833846989));
#21074=CARTESIAN_POINT('',(43.9750046174461,7.92280378598205,-47.0072401194241));
#21075=CARTESIAN_POINT('Ctrl Pts',(43.9750046174461,7.92280378598205,-47.0072401194241));
#21076=CARTESIAN_POINT('Ctrl Pts',(44.0191184364596,7.90807633871839,-47.1700481506604));
#21077=CARTESIAN_POINT('Ctrl Pts',(44.0399563324054,7.89944521405426,-47.3379114457046));
#21078=CARTESIAN_POINT('Ctrl Pts',(44.0399563324054,7.89944521405426,-47.6620885542954));
#21079=CARTESIAN_POINT('Ctrl Pts',(44.0191184364596,7.9080763387184,-47.8299518493397));
#21080=CARTESIAN_POINT('Ctrl Pts',(43.9750046174461,7.92280378598205,-47.9927598805759));
#21081=CARTESIAN_POINT('Ctrl Pts',(43.5,8.,-46.2048166153011));
#21082=CARTESIAN_POINT('Ctrl Pts',(43.7266147755088,8.,-46.4235257747395));
#21083=CARTESIAN_POINT('Ctrl Pts',(43.8929060558365,7.95021248156921,-46.704244244619));
#21084=CARTESIAN_POINT('Ctrl Pts',(43.9750046174461,7.92280378598205,-47.0072401194241));
#21085=CARTESIAN_POINT('Origin',(43.5,6.5,-40.5));
#21086=CARTESIAN_POINT('Origin',(3.99999999999999,-1.5,-55.));
#21087=CARTESIAN_POINT('Origin',(24.5,7.75,-40.25));
#21088=CARTESIAN_POINT('',(4.,7.5,-40.));
#21089=CARTESIAN_POINT('',(24.5,7.5,-40.));
#21090=CARTESIAN_POINT('',(3.5,8.,-40.5));
#21091=CARTESIAN_POINT('Origin',(24.5,7.75,-40.25));
#21092=CARTESIAN_POINT('',(-16.,7.5,-40.));
#21093=CARTESIAN_POINT('',(-16.5,8.,-40.5));
#21094=CARTESIAN_POINT('',(24.5,7.5,-40.));
#21095=CARTESIAN_POINT('Origin',(-16.25,7.75,-47.5));
#21096=CARTESIAN_POINT('',(-16.,7.5,-47.5));
#21097=CARTESIAN_POINT('',(-16.5,8.,-38.));
#21098=CARTESIAN_POINT('Origin',(24.5,7.75,-40.25));
#21099=CARTESIAN_POINT('',(-35.5,7.5,-40.));
#21100=CARTESIAN_POINT('',(-35.5,8.,-40.5));
#21101=CARTESIAN_POINT('',(24.5,7.5,-40.));
#21102=CARTESIAN_POINT('Origin',(-35.5,6.5,-40.25));
#21103=CARTESIAN_POINT('',(-37.,6.5,-40.5));
#21104=CARTESIAN_POINT('Origin',(-35.5,6.5,-40.5));
#21105=CARTESIAN_POINT('',(-36.5,6.5,-40.));
#21106=CARTESIAN_POINT('',(-37.,6.5,-40.5));
#21107=CARTESIAN_POINT('Origin',(-35.5,6.5,-40.));
#21108=CARTESIAN_POINT('Origin',(-36.75,3.25,-40.25));
#21109=CARTESIAN_POINT('',(-37.,-9.5,-40.5));
#21110=CARTESIAN_POINT('',(-36.5,-9.5,-40.));
#21111=CARTESIAN_POINT('',(-37.,-9.5,-40.5));
#21112=CARTESIAN_POINT('',(-36.5,3.25,-40.));
#21113=CARTESIAN_POINT('',(-37.,3.25,-40.5));
#21114=CARTESIAN_POINT('Origin',(-35.5,-9.5,-40.25));
#21115=CARTESIAN_POINT('',(-35.5,-11.,-40.5));
#21116=CARTESIAN_POINT('Origin',(-35.5,-9.5,-40.5));
#21117=CARTESIAN_POINT('',(-35.5,-10.5,-40.));
#21118=CARTESIAN_POINT('',(-35.5,-11.,-40.5));
#21119=CARTESIAN_POINT('Origin',(-35.5,-9.5,-40.));
#21120=CARTESIAN_POINT('Origin',(-16.5,-10.75,-40.25));
#21121=CARTESIAN_POINT('',(43.5,-10.5,-40.));
#21122=CARTESIAN_POINT('',(43.5,-11.,-40.5));
#21123=CARTESIAN_POINT('',(-16.5,-10.5,-40.));
#21124=CARTESIAN_POINT('',(-16.5,-11.,-40.5));
#21125=CARTESIAN_POINT('Origin',(43.5,-9.5,-40.25));
#21126=CARTESIAN_POINT('',(44.5,-9.5,-40.));
#21127=CARTESIAN_POINT('',(45.,-9.5,-40.5));
#21128=CARTESIAN_POINT('Origin',(43.5,-9.5,-40.));
#21129=CARTESIAN_POINT('Origin',(44.75,-6.25,-40.25));
#21130=CARTESIAN_POINT('',(44.5,6.5,-40.));
#21131=CARTESIAN_POINT('',(45.,6.5,-40.5));
#21132=CARTESIAN_POINT('',(44.5,-6.25,-40.));
#21133=CARTESIAN_POINT('Origin',(43.5,6.5,-40.25));
#21134=CARTESIAN_POINT('',(43.5,7.5,-40.));
#21135=CARTESIAN_POINT('',(43.5,8.,-40.5));
#21136=CARTESIAN_POINT('Origin',(43.5,6.5,-40.));
#21137=CARTESIAN_POINT('Origin',(24.5,7.75,-40.25));
#21138=CARTESIAN_POINT('',(24.5,7.5,-40.));
#21139=CARTESIAN_POINT('',(21.5,8.,-40.5));
#21140=CARTESIAN_POINT('Origin',(21.75,7.75,-47.5));
#21141=CARTESIAN_POINT('',(21.5,8.,-38.));
#21142=CARTESIAN_POINT('Origin',(12.5,7.75,-37.75));
#21143=CARTESIAN_POINT('',(12.5,7.5,-37.5));
#21144=CARTESIAN_POINT('Origin',(31.5,7.75,-37.75));
#21145=CARTESIAN_POINT('',(31.5,7.5,-37.5));
#21146=CARTESIAN_POINT('Origin',(3.75,7.75,-47.5));
#21147=CARTESIAN_POINT('',(4.,7.5,-47.5));
#21148=CARTESIAN_POINT('',(3.5,8.,-38.));
#21149=CARTESIAN_POINT('Origin',(22.5,7.75,-37.75));
#21150=CARTESIAN_POINT('',(22.5,7.5,-37.5));
#21151=CARTESIAN_POINT('Origin',(-37.,-11.,-55.));
#21152=CARTESIAN_POINT('',(-35.5,-11.,-55.));
#21153=CARTESIAN_POINT('Origin',(-35.5,-9.5,-55.));
#21154=CARTESIAN_POINT('',(-37.,-9.5,-55.));
#21155=CARTESIAN_POINT('Origin',(-37.,8.,-55.));
#21156=CARTESIAN_POINT('',(-37.,6.5,-55.));
#21157=CARTESIAN_POINT('Origin',(-35.5,6.5,-55.));
#21158=CARTESIAN_POINT('',(-35.9750046174461,7.92280378598206,-47.0072401194241));
#21159=CARTESIAN_POINT('Ctrl Pts',(-35.9750046174461,7.92280378598206,-47.0072401194241));
#21160=CARTESIAN_POINT('Ctrl Pts',(-35.8929060558365,7.95021248156921,-46.704244244619));
#21161=CARTESIAN_POINT('Ctrl Pts',(-35.7266147755088,8.,-46.4235257747395));
#21162=CARTESIAN_POINT('Ctrl Pts',(-35.5,8.,-46.2048166153011));
#21163=CARTESIAN_POINT('',(-35.9750046174461,7.92280378598205,-47.9927598805758));
#21164=CARTESIAN_POINT('Ctrl Pts',(-35.9750046174461,7.92280378598205,-47.9927598805758));
#21165=CARTESIAN_POINT('Ctrl Pts',(-36.0191184364596,7.90807633871838,-47.8299518493395));
#21166=CARTESIAN_POINT('Ctrl Pts',(-36.0399563352666,7.8994452073828,-47.662088554661));
#21167=CARTESIAN_POINT('Ctrl Pts',(-36.0399563352666,7.8994452073828,-47.337911445339));
#21168=CARTESIAN_POINT('Ctrl Pts',(-36.0191184364596,7.90807633871839,-47.1700481506605));
#21169=CARTESIAN_POINT('Ctrl Pts',(-35.9750046174461,7.92280378598206,-47.0072401194241));
#21170=CARTESIAN_POINT('Ctrl Pts',(-35.5,8.,-48.7951833846989));
#21171=CARTESIAN_POINT('Ctrl Pts',(-35.7266147755088,8.,-48.5764742252605));
#21172=CARTESIAN_POINT('Ctrl Pts',(-35.8929060558365,7.95021248156921,-48.295755755381));
#21173=CARTESIAN_POINT('Ctrl Pts',(-35.9750046174461,7.92280378598205,-47.9927598805758));
#21174=CARTESIAN_POINT('Origin',(4.,2.,-40.));
#21175=CARTESIAN_POINT('',(4.,0.25,-40.));
#21176=CARTESIAN_POINT('Origin',(0.,5.,-37.5));
#21177=CARTESIAN_POINT('Origin',(3.99999999999999,-1.5,-40.));
#21178=CARTESIAN_POINT('',(-16.,0.25,-40.));
#21179=CARTESIAN_POINT('Origin',(-16.,2.,-40.));
#21180=CARTESIAN_POINT('Origin',(-20.,5.,-37.5));
#21181=CARTESIAN_POINT('Ctrl Pts',(43.9750046174461,7.92280378598205,-47.9927598805759));
#21182=CARTESIAN_POINT('Ctrl Pts',(44.0191184364596,7.9080763387184,-47.8299518493397));
#21183=CARTESIAN_POINT('Ctrl Pts',(44.0399563324054,7.89944521405426,-47.6620885542954));
#21184=CARTESIAN_POINT('Ctrl Pts',(44.0399563324054,7.89944521405426,-47.3379114457046));
#21185=CARTESIAN_POINT('Ctrl Pts',(44.0191184364596,7.90807633871839,-47.1700481506604));
#21186=CARTESIAN_POINT('Ctrl Pts',(43.9750046174461,7.92280378598205,-47.0072401194241));
#21187=CARTESIAN_POINT('Ctrl Pts',(43.8166697449641,7.7818691906547,-47.947530394193));
#21188=CARTESIAN_POINT('Ctrl Pts',(43.8570720539749,7.77209665345059,-47.8007056846591));
#21189=CARTESIAN_POINT('Ctrl Pts',(43.8766475282555,7.76602646568173,-47.6477355606756));
#21190=CARTESIAN_POINT('Ctrl Pts',(43.8766475282555,7.76602646568173,-47.3522644393244));
#21191=CARTESIAN_POINT('Ctrl Pts',(43.857072053975,7.77209665345058,-47.199294315341));
#21192=CARTESIAN_POINT('Ctrl Pts',(43.8166697449641,7.7818691906547,-47.052469605807));
#21193=CARTESIAN_POINT('Ctrl Pts',(43.658334872482,7.64093459532735,-47.9023009078101));
#21194=CARTESIAN_POINT('Ctrl Pts',(43.6948644867881,7.63597968526781,-47.7714312414787));
#21195=CARTESIAN_POINT('Ctrl Pts',(43.71331135762,7.63258420254192,-47.6333822918808));
#21196=CARTESIAN_POINT('Ctrl Pts',(43.71331135762,7.63258420254192,-47.3666177081192));
#21197=CARTESIAN_POINT('Ctrl Pts',(43.6948644867881,7.63597968526781,-47.2285687585214));
#21198=CARTESIAN_POINT('Ctrl Pts',(43.658334872482,7.64093459532735,-47.0976990921899));
#21199=CARTESIAN_POINT('Ctrl Pts',(43.5,7.5,-47.8570714214271));
#21200=CARTESIAN_POINT('Ctrl Pts',(43.5328181043034,7.5,-47.742185076798));
#21201=CARTESIAN_POINT('Ctrl Pts',(43.5500025534701,7.49916545416939,-47.619029298261));
#21202=CARTESIAN_POINT('Ctrl Pts',(43.5500025534701,7.49916545416939,-47.380970701739));
#21203=CARTESIAN_POINT('Ctrl Pts',(43.5328181043035,7.5,-47.2578149232021));
#21204=CARTESIAN_POINT('Ctrl Pts',(43.5,7.5,-47.1429285785729));
#21205=CARTESIAN_POINT('',(43.5,7.5,-47.1429285785729));
#21206=CARTESIAN_POINT('',(43.5,7.5,-47.1429285785729));
#21207=CARTESIAN_POINT('',(43.5,7.5,-47.8570714214271));
#21208=CARTESIAN_POINT('',(43.9750046174461,7.92280378598205,-47.9927598805759));
#21209=CARTESIAN_POINT('Ctrl Pts',(43.5,7.5,-47.8570714214271));
#21210=CARTESIAN_POINT('Ctrl Pts',(43.5328181043034,7.5,-47.742185076798));
#21211=CARTESIAN_POINT('Ctrl Pts',(43.5500025534701,7.49916545416939,-47.619029298261));
#21212=CARTESIAN_POINT('Ctrl Pts',(43.5500025534701,7.49916545416939,-47.380970701739));
#21213=CARTESIAN_POINT('Ctrl Pts',(43.5328181043035,7.5,-47.2578149232021));
#21214=CARTESIAN_POINT('Ctrl Pts',(43.5,7.5,-47.1429285785729));
#21215=CARTESIAN_POINT('Origin',(42.25,7.75,-47.5));
#21216=CARTESIAN_POINT('',(43.1527777777778,7.5,-46.5645897777175));
#21217=CARTESIAN_POINT('',(43.5,8.,-46.2048166153011));
#21218=CARTESIAN_POINT('',(40.95,7.5,-47.5));
#21219=CARTESIAN_POINT('Origin',(42.25,7.5,-47.5));
#21220=CARTESIAN_POINT('',(43.1527777777778,7.5,-48.4354102222825));
#21221=CARTESIAN_POINT('Origin',(42.25,7.5,-47.5));
#21222=CARTESIAN_POINT('',(43.1527777777778,7.5,-48.4354102222825));
#21223=CARTESIAN_POINT('Ctrl Pts',(43.9750046174461,7.92280378598205,-47.0072401194241));
#21224=CARTESIAN_POINT('Ctrl Pts',(43.8929060558365,7.95021248156921,-46.704244244619));
#21225=CARTESIAN_POINT('Ctrl Pts',(43.7266147755088,8.,-46.4235257747395));
#21226=CARTESIAN_POINT('Ctrl Pts',(43.5,8.,-46.2048166153011));
#21227=CARTESIAN_POINT('Ctrl Pts',(43.8166697449641,7.7818691906547,-47.052469605807));
#21228=CARTESIAN_POINT('Ctrl Pts',(43.7411120931071,7.80014165437948,-46.7775693027908));
#21229=CARTESIAN_POINT('Ctrl Pts',(43.5898911851839,7.83333333333333,-46.5231993141155));
#21230=CARTESIAN_POINT('Ctrl Pts',(43.3842592592593,7.83333333333333,-46.3247410027733));
#21231=CARTESIAN_POINT('Ctrl Pts',(43.658334872482,7.64093459532735,-47.0976990921899));
#21232=CARTESIAN_POINT('Ctrl Pts',(43.5893181303776,7.65007082718974,-46.8508943609626));
#21233=CARTESIAN_POINT('Ctrl Pts',(43.453167594859,7.66666666666667,-46.6228728534914));
#21234=CARTESIAN_POINT('Ctrl Pts',(43.2685185185185,7.66666666666667,-46.4446653902454));
#21235=CARTESIAN_POINT('Ctrl Pts',(43.5,7.5,-47.1429285785729));
#21236=CARTESIAN_POINT('Ctrl Pts',(43.4375241676482,7.5,-46.9242194191345));
#21237=CARTESIAN_POINT('Ctrl Pts',(43.3164440045341,7.5,-46.7225463928674));
#21238=CARTESIAN_POINT('Ctrl Pts',(43.1527777777778,7.5,-46.5645897777175));
#21239=CARTESIAN_POINT('Ctrl Pts',(43.5,7.5,-47.1429285785729));
#21240=CARTESIAN_POINT('Ctrl Pts',(43.4375241676482,7.5,-46.9242194191345));
#21241=CARTESIAN_POINT('Ctrl Pts',(43.3164440045341,7.5,-46.7225463928674));
#21242=CARTESIAN_POINT('Ctrl Pts',(43.1527777777778,7.5,-46.5645897777175));
#21243=CARTESIAN_POINT('Ctrl Pts',(43.5,8.,-48.7951833846989));
#21244=CARTESIAN_POINT('Ctrl Pts',(43.7266147755088,8.,-48.5764742252605));
#21245=CARTESIAN_POINT('Ctrl Pts',(43.8929060558365,7.95021248156921,-48.295755755381));
#21246=CARTESIAN_POINT('Ctrl Pts',(43.9750046174461,7.92280378598205,-47.9927598805759));
#21247=CARTESIAN_POINT('Ctrl Pts',(43.3842592592593,7.83333333333333,-48.6752589972267));
#21248=CARTESIAN_POINT('Ctrl Pts',(43.5898911851839,7.83333333333333,-48.4768006858845));
#21249=CARTESIAN_POINT('Ctrl Pts',(43.7411120931071,7.80014165437948,-48.2224306972092));
#21250=CARTESIAN_POINT('Ctrl Pts',(43.8166697449641,7.7818691906547,-47.947530394193));
#21251=CARTESIAN_POINT('Ctrl Pts',(43.2685185185185,7.66666666666667,-48.5553346097546));
#21252=CARTESIAN_POINT('Ctrl Pts',(43.453167594859,7.66666666666667,-48.3771271465086));
#21253=CARTESIAN_POINT('Ctrl Pts',(43.5893181303776,7.65007082718974,-48.1491056390374));
#21254=CARTESIAN_POINT('Ctrl Pts',(43.658334872482,7.64093459532735,-47.9023009078101));
#21255=CARTESIAN_POINT('Ctrl Pts',(43.1527777777778,7.5,-48.4354102222825));
#21256=CARTESIAN_POINT('Ctrl Pts',(43.3164440045341,7.5,-48.2774536071326));
#21257=CARTESIAN_POINT('Ctrl Pts',(43.4375241676482,7.5,-48.0757805808655));
#21258=CARTESIAN_POINT('Ctrl Pts',(43.5,7.5,-47.8570714214271));
#21259=CARTESIAN_POINT('Ctrl Pts',(43.1527777777778,7.5,-48.4354102222825));
#21260=CARTESIAN_POINT('Ctrl Pts',(43.3164440045341,7.5,-48.2774536071326));
#21261=CARTESIAN_POINT('Ctrl Pts',(43.4375241676482,7.5,-48.0757805808655));
#21262=CARTESIAN_POINT('Ctrl Pts',(43.5,7.5,-47.8570714214271));
#21263=CARTESIAN_POINT('Origin',(42.25,8.,-47.5));
#21264=CARTESIAN_POINT('',(40.95,0.,-47.5));
#21265=CARTESIAN_POINT('',(40.95,8.,-47.5));
#21266=CARTESIAN_POINT('Origin',(42.25,0.,-47.5));
#21267=CARTESIAN_POINT('Ctrl Pts',(-35.9750046174461,7.92280378598206,-47.0072401194241));
#21268=CARTESIAN_POINT('Ctrl Pts',(-36.0191184364596,7.90807633871839,-47.1700481506605));
#21269=CARTESIAN_POINT('Ctrl Pts',(-36.0399563352666,7.8994452073828,-47.337911445339));
#21270=CARTESIAN_POINT('Ctrl Pts',(-36.0399563352666,7.8994452073828,-47.662088554661));
#21271=CARTESIAN_POINT('Ctrl Pts',(-36.0191184364596,7.90807633871838,-47.8299518493395));
#21272=CARTESIAN_POINT('Ctrl Pts',(-35.9750046174461,7.92280378598205,-47.9927598805758));
#21273=CARTESIAN_POINT('Ctrl Pts',(-35.8166697449641,7.78186919065471,-47.0524696058071));
#21274=CARTESIAN_POINT('Ctrl Pts',(-35.857072053975,7.77209665345057,-47.1992943153412));
#21275=CARTESIAN_POINT('Ctrl Pts',(-35.8766475311167,7.76602645901027,-47.3522644389587));
#21276=CARTESIAN_POINT('Ctrl Pts',(-35.8766475311167,7.76602645901027,-47.6477355610413));
#21277=CARTESIAN_POINT('Ctrl Pts',(-35.857072053975,7.77209665345057,-47.8007056846588));
#21278=CARTESIAN_POINT('Ctrl Pts',(-35.8166697449641,7.7818691906547,-47.9475303941929));
#21279=CARTESIAN_POINT('Ctrl Pts',(-35.658334872482,7.64093459532735,-47.09769909219));
#21280=CARTESIAN_POINT('Ctrl Pts',(-35.6948644867881,7.63597968526782,-47.2285687585214));
#21281=CARTESIAN_POINT('Ctrl Pts',(-35.7133113651929,7.63258419989791,-47.3666177074644));
#21282=CARTESIAN_POINT('Ctrl Pts',(-35.7133113651929,7.63258419989791,-47.6333822925356));
#21283=CARTESIAN_POINT('Ctrl Pts',(-35.6948644867881,7.63597968526782,-47.7714312414786));
#21284=CARTESIAN_POINT('Ctrl Pts',(-35.6583348724821,7.64093459532735,-47.90230090781));
#21285=CARTESIAN_POINT('Ctrl Pts',(-35.5,7.5,-47.1429285785729));
#21286=CARTESIAN_POINT('Ctrl Pts',(-35.5328181043034,7.5,-47.2578149232021));
#21287=CARTESIAN_POINT('Ctrl Pts',(-35.550002561043,7.49916545152538,-47.3809707010842));
#21288=CARTESIAN_POINT('Ctrl Pts',(-35.550002561043,7.49916545152537,-47.6190292989158));
#21289=CARTESIAN_POINT('Ctrl Pts',(-35.5328181043034,7.5,-47.7421850767979));
#21290=CARTESIAN_POINT('Ctrl Pts',(-35.5,7.5,-47.8570714214271));
#21291=CARTESIAN_POINT('',(-35.5,7.5,-47.8570714214271));
#21292=CARTESIAN_POINT('',(-35.5,7.5,-47.8570714214271));
#21293=CARTESIAN_POINT('',(-35.5,7.5,-47.1429285785729));
#21294=CARTESIAN_POINT('',(-35.9750046174461,7.92280378598206,-47.0072401194241));
#21295=CARTESIAN_POINT('',(-35.550002561043,7.49916545152538,-47.5));
#21296=CARTESIAN_POINT('Ctrl Pts',(-35.5,7.5,-47.1429285785729));
#21297=CARTESIAN_POINT('Ctrl Pts',(-35.5328181043034,7.5,-47.2578149232021));
#21298=CARTESIAN_POINT('Ctrl Pts',(-35.550002561043,7.49916545152538,-47.3809707010842));
#21299=CARTESIAN_POINT('Ctrl Pts',(-35.550002561043,7.49916545152538,-47.5));
#21300=CARTESIAN_POINT('Ctrl Pts',(-35.550002561043,7.49916545152538,-47.5));
#21301=CARTESIAN_POINT('Ctrl Pts',(-35.550002561043,7.49916545152537,-47.6190292989158));
#21302=CARTESIAN_POINT('Ctrl Pts',(-35.5328181043034,7.5,-47.7421850767979));
#21303=CARTESIAN_POINT('Ctrl Pts',(-35.5,7.5,-47.8570714214271));
#21304=CARTESIAN_POINT('Origin',(-34.25,7.75,-47.5));
#21305=CARTESIAN_POINT('',(-35.1527777777778,7.5,-48.4354102222825));
#21306=CARTESIAN_POINT('',(-35.5,8.,-48.7951833846989));
#21307=CARTESIAN_POINT('',(-35.1527777777778,7.5,-46.5645897777175));
#21308=CARTESIAN_POINT('Origin',(-34.25,7.5,-47.5));
#21309=CARTESIAN_POINT('',(-35.1527777777778,7.5,-46.5645897777175));
#21310=CARTESIAN_POINT('Ctrl Pts',(-35.9750046174461,7.92280378598205,-47.9927598805758));
#21311=CARTESIAN_POINT('Ctrl Pts',(-35.8929060558365,7.95021248156921,-48.295755755381));
#21312=CARTESIAN_POINT('Ctrl Pts',(-35.7266147755088,8.,-48.5764742252605));
#21313=CARTESIAN_POINT('Ctrl Pts',(-35.5,8.,-48.7951833846989));
#21314=CARTESIAN_POINT('Ctrl Pts',(-35.8166697449641,7.7818691906547,-47.9475303941929));
#21315=CARTESIAN_POINT('Ctrl Pts',(-35.7411120931071,7.80014165437948,-48.2224306972092));
#21316=CARTESIAN_POINT('Ctrl Pts',(-35.5898911851839,7.83333333333334,-48.4768006858845));
#21317=CARTESIAN_POINT('Ctrl Pts',(-35.3842592592593,7.83333333333333,-48.6752589972267));
#21318=CARTESIAN_POINT('Ctrl Pts',(-35.6583348724821,7.64093459532735,-47.90230090781));
#21319=CARTESIAN_POINT('Ctrl Pts',(-35.5893181303776,7.65007082718974,-48.1491056390373));
#21320=CARTESIAN_POINT('Ctrl Pts',(-35.453167594859,7.66666666666667,-48.3771271465086));
#21321=CARTESIAN_POINT('Ctrl Pts',(-35.2685185185185,7.66666666666667,-48.5553346097546));
#21322=CARTESIAN_POINT('Ctrl Pts',(-35.5,7.5,-47.8570714214271));
#21323=CARTESIAN_POINT('Ctrl Pts',(-35.4375241676482,7.5,-48.0757805808655));
#21324=CARTESIAN_POINT('Ctrl Pts',(-35.3164440045342,7.5,-48.2774536071326));
#21325=CARTESIAN_POINT('Ctrl Pts',(-35.1527777777778,7.5,-48.4354102222825));
#21326=CARTESIAN_POINT('Ctrl Pts',(-35.5,7.5,-47.8570714214271));
#21327=CARTESIAN_POINT('Ctrl Pts',(-35.4375241676482,7.5,-48.0757805808655));
#21328=CARTESIAN_POINT('Ctrl Pts',(-35.3164440045342,7.5,-48.2774536071326));
#21329=CARTESIAN_POINT('Ctrl Pts',(-35.1527777777778,7.5,-48.4354102222825));
#21330=CARTESIAN_POINT('Ctrl Pts',(-35.5,8.,-46.2048166153011));
#21331=CARTESIAN_POINT('Ctrl Pts',(-35.7266147755088,8.,-46.4235257747395));
#21332=CARTESIAN_POINT('Ctrl Pts',(-35.8929060558365,7.95021248156921,-46.704244244619));
#21333=CARTESIAN_POINT('Ctrl Pts',(-35.9750046174461,7.92280378598206,-47.0072401194241));
#21334=CARTESIAN_POINT('Ctrl Pts',(-35.3842592592593,7.83333333333333,-46.3247410027733));
#21335=CARTESIAN_POINT('Ctrl Pts',(-35.5898911851839,7.83333333333333,-46.5231993141155));
#21336=CARTESIAN_POINT('Ctrl Pts',(-35.7411120931071,7.80014165437948,-46.7775693027908));
#21337=CARTESIAN_POINT('Ctrl Pts',(-35.8166697449641,7.7818691906547,-47.0524696058071));
#21338=CARTESIAN_POINT('Ctrl Pts',(-35.2685185185185,7.66666666666667,-46.4446653902454));
#21339=CARTESIAN_POINT('Ctrl Pts',(-35.4531675948591,7.66666666666667,-46.6228728534915));
#21340=CARTESIAN_POINT('Ctrl Pts',(-35.5893181303776,7.65007082718974,-46.8508943609627));
#21341=CARTESIAN_POINT('Ctrl Pts',(-35.658334872482,7.64093459532735,-47.09769909219));
#21342=CARTESIAN_POINT('Ctrl Pts',(-35.1527777777778,7.5,-46.5645897777175));
#21343=CARTESIAN_POINT('Ctrl Pts',(-35.3164440045342,7.5,-46.7225463928674));
#21344=CARTESIAN_POINT('Ctrl Pts',(-35.4375241676482,7.5,-46.9242194191345));
#21345=CARTESIAN_POINT('Ctrl Pts',(-35.5,7.5,-47.1429285785729));
#21346=CARTESIAN_POINT('Ctrl Pts',(-35.1527777777778,7.5,-46.5645897777175));
#21347=CARTESIAN_POINT('Ctrl Pts',(-35.3164440045342,7.5,-46.7225463928674));
#21348=CARTESIAN_POINT('Ctrl Pts',(-35.4375241676482,7.5,-46.9242194191345));
#21349=CARTESIAN_POINT('Ctrl Pts',(-35.5,7.5,-47.1429285785729));
#21350=CARTESIAN_POINT('Origin',(-34.25,8.,-47.5));
#21351=CARTESIAN_POINT('',(-35.55,0.,-47.5));
#21352=CARTESIAN_POINT('',(-35.55,8.,-47.5));
#21353=CARTESIAN_POINT('Origin',(-34.25,0.,-47.5));
#21354=CARTESIAN_POINT('Origin',(44.75,-3.,-47.5));
#21355=CARTESIAN_POINT('',(44.5,-3.,-45.));
#21356=CARTESIAN_POINT('',(44.75,-3.,-44.75));
#21357=CARTESIAN_POINT('Origin',(44.5,-3.,-47.5));
#21358=CARTESIAN_POINT('Origin',(45.,-3.,-47.5));
#21359=CARTESIAN_POINT('',(40.,-3.,-45.));
#21360=CARTESIAN_POINT('',(45.,-3.,-45.));
#21361=CARTESIAN_POINT('Origin',(40.,-3.,-47.5));
#21362=CARTESIAN_POINT('Origin',(39.75,-3.,-47.5));
#21363=CARTESIAN_POINT('',(39.5,-3.,-44.5));
#21364=CARTESIAN_POINT('Origin',(39.5,-3.,-47.5));
#21365=CARTESIAN_POINT('',(39.75,-3.,-44.75));
#21366=CARTESIAN_POINT('Origin',(39.5,8.,-53.));
#21367=CARTESIAN_POINT('',(39.5,-9.,-42.));
#21368=CARTESIAN_POINT('',(39.5,-9.,-53.));
#21369=CARTESIAN_POINT('',(39.5,8.,-42.));
#21370=CARTESIAN_POINT('Origin',(-34.25,0.,-47.5));
#21371=CARTESIAN_POINT('Origin',(42.25,0.,-47.5));
#21372=CARTESIAN_POINT('Origin',(-25.2,-3.55,-30.9504065443768));
#21373=CARTESIAN_POINT('',(-25.2,-3.55,-30.9504065443768));
#21374=CARTESIAN_POINT('Origin',(-25.2,-3.55,-35.0495934556232));
#21375=CARTESIAN_POINT('',(-25.2,-3.55,-35.0495934556232));
#21376=CARTESIAN_POINT('Origin',(-25.2,-5.55111512312578E-16,-37.0991869112463));
#21377=CARTESIAN_POINT('Origin',(25.2,-3.55,-35.0495934556232));
#21378=CARTESIAN_POINT('',(25.2,-3.55,-35.0495934556232));
#21379=CARTESIAN_POINT('Origin',(25.2,-3.55,-30.9504065443768));
#21380=CARTESIAN_POINT('',(25.2,-3.55,-30.9504065443768));
#21381=CARTESIAN_POINT('Origin',(25.2,2.51002806498228E-16,-28.9008130887537));
#21382=CARTESIAN_POINT('Origin',(39.5,8.,-42.));
#21383=CARTESIAN_POINT('',(39.5,-9.,-42.));
#21384=CARTESIAN_POINT('Origin',(4.,-9.,-47.5));
#21385=CARTESIAN_POINT('Origin',(18.,5.,-37.5));
#37155=UNCERTAINTY_MEASURE_WITH_UNIT(LENGTH_MEASURE(0.01),#37182,
'DISTANCE_ACCURACY_VALUE',
'Maximum model space distance between geometric entities at asserted c
onnectivities');
#37166=UNCERTAINTY_MEASURE_WITH_UNIT(LENGTH_MEASURE(0.01),#37182,
'DISTANCE_ACCURACY_VALUE',
'Maximum model space distance between geometric entities at asserted c
onnectivities');
#37170=(
GEOMETRIC_REPRESENTATION_CONTEXT(3)
GLOBAL_UNCERTAINTY_ASSIGNED_CONTEXT((#37155))
GLOBAL_UNIT_ASSIGNED_CONTEXT((#37182,#37184,#37185))
REPRESENTATION_CONTEXT('','3D')
);
#37181=(
GEOMETRIC_REPRESENTATION_CONTEXT(3)
GLOBAL_UNCERTAINTY_ASSIGNED_CONTEXT((#37166))
GLOBAL_UNIT_ASSIGNED_CONTEXT((#37182,#37184,#37185))
REPRESENTATION_CONTEXT('','3D')
);
#37182=(
LENGTH_UNIT()
NAMED_UNIT(*)
SI_UNIT(.MILLI.,.METRE.)
);
#37184=(
NAMED_UNIT(*)
PLANE_ANGLE_UNIT()
SI_UNIT($,.RADIAN.)
);
#37185=(
NAMED_UNIT(*)
SI_UNIT($,.STERADIAN.)
SOLID_ANGLE_UNIT()
);
#37189=SHAPE_DEFINITION_REPRESENTATION(#37203,#37240);
#37203=PRODUCT_DEFINITION_SHAPE('',$,#37255);
#37240=SHAPE_REPRESENTATION('',(#15137),#37170);
#37251=PRODUCT_DEFINITION_CONTEXT('part definition',#37295,'design');
#37255=PRODUCT_DEFINITION('2026-10-20-13-23-49-638',
'03_Camera_Housing_Body_PLA',#37269,#37251);
#37269=PRODUCT_DEFINITION_FORMATION('',$,#37300);
#37295=APPLICATION_CONTEXT(
'Core Data for Automotive Mechanical Design Process');
#37296=PRODUCT_CONTEXT('part definition',#37295,'mechanical');
#37300=PRODUCT('2026-10-20-13-23-49-638','03_Camera_Housing_Body_PLA',$,
(#37296));
#37346=COLOUR_RGB('Dark Blue',0.08,0.2,0.34);
#37347=FILL_AREA_STYLE_COLOUR('',#37346);
#37348=FILL_AREA_STYLE('',(#37347));
#37349=SURFACE_STYLE_FILL_AREA(#37348);
#37350=SURFACE_SIDE_STYLE('',(#37349));
#37351=SURFACE_STYLE_USAGE(.BOTH.,#37350);
#37352=PRESENTATION_STYLE_ASSIGNMENT((#37351));
ENDSEC;
END-ISO-10303-21;
